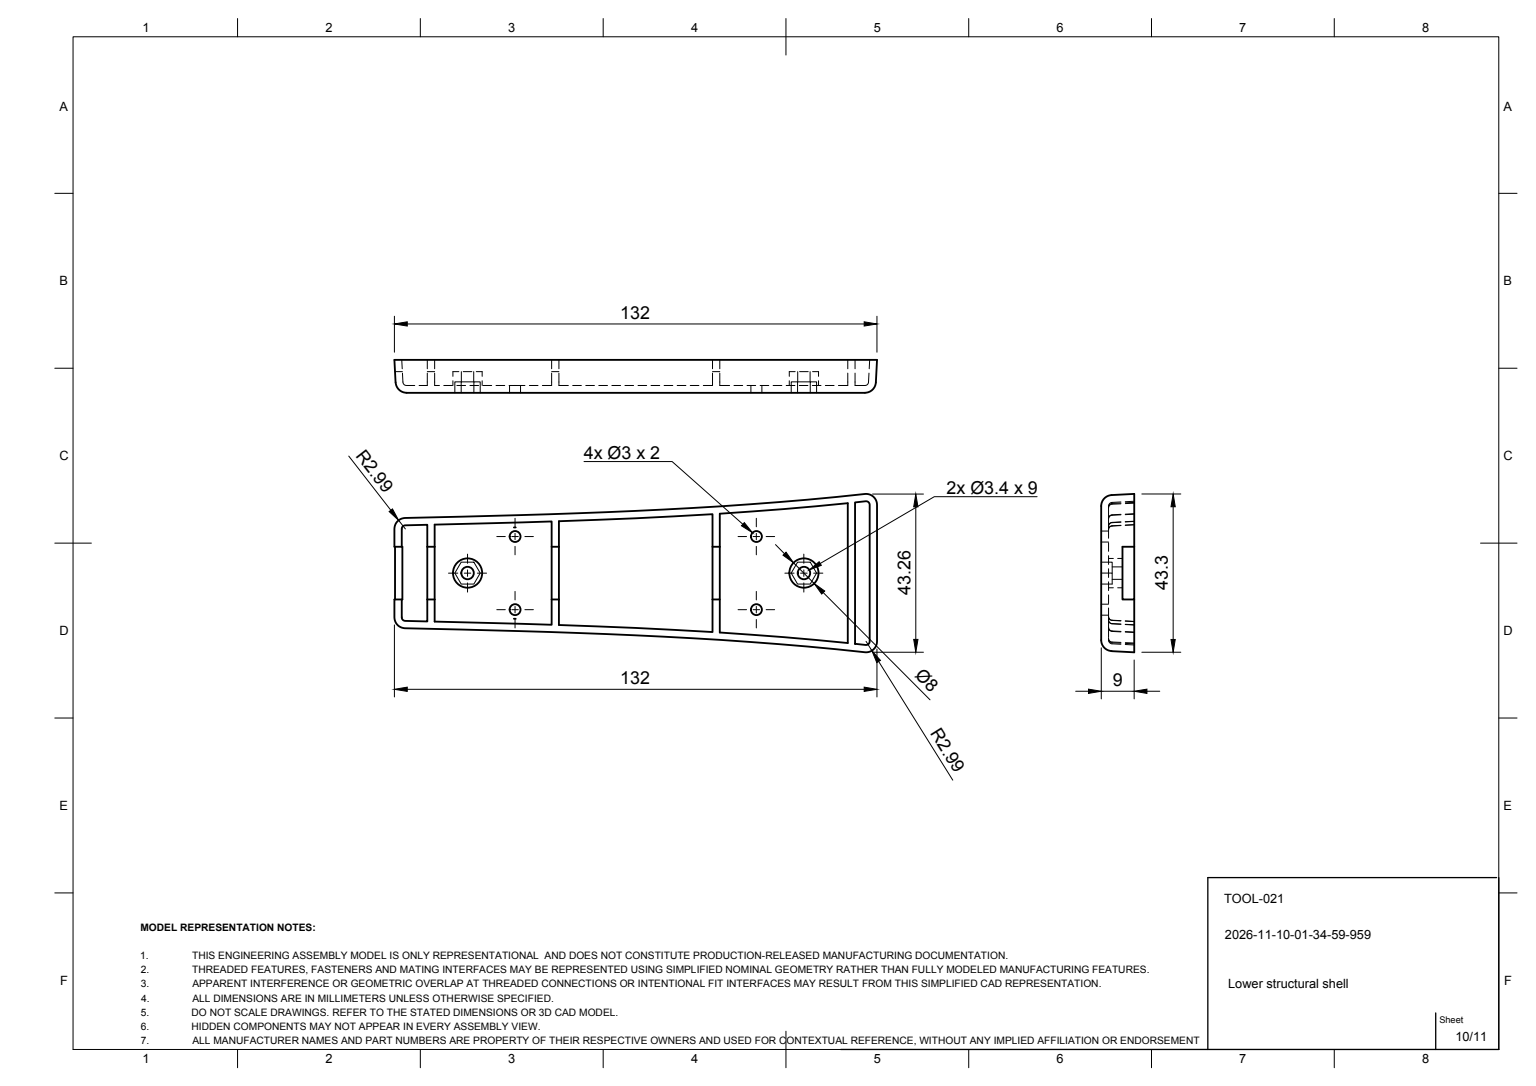
ISO-10303-21;
HEADER;
/* Generated by software containing ST-Developer
 * from STEP Tools, Inc. (www.steptools.com) 
 */

FILE_DESCRIPTION(
/* description */ (''),
/* implementation_level */ '2;1');

FILE_NAME(
/* name */ 'Lower structural shell.step',
/* time_stamp */ '2026-11-10T09:05:57-08:00',
/* author */ (''),
/* organization */ (''),
/* preprocessor_version */ 'ST-DEVELOPER v20.2',
/* originating_system */ 'Autodesk Translation Framework v15.17.0.0',
/* authorisation */ '');

FILE_SCHEMA (('AUTOMOTIVE_DESIGN { 1 0 10303 214 3 1 1 }'));
ENDSEC;

DATA;
#10=MECHANICAL_DESIGN_GEOMETRIC_PRESENTATION_REPRESENTATION('',(#570),#19618);
#83=SPHERICAL_SURFACE('',#7546,0.0999999999999999);
#84=SPHERICAL_SURFACE('',#7549,0.0999999999999997);
#85=SPHERICAL_SURFACE('',#7553,0.0999999999999998);
#86=SPHERICAL_SURFACE('',#7557,0.1);
#87=SPHERICAL_SURFACE('',#7562,0.3);
#88=SPHERICAL_SURFACE('',#7566,0.3);
#89=SPHERICAL_SURFACE('',#7570,0.3);
#90=SPHERICAL_SURFACE('',#7575,0.3);
#123=B_SPLINE_SURFACE_WITH_KNOTS('',3,3,((#12819,#12820,#12821,#12822),
(#12823,#12824,#12825,#12826),(#12827,#12828,#12829,#12830),(#12831,#12832,
#12833,#12834)),.UNSPECIFIED.,.F.,.F.,.F.,(4,4),(4,4),(0.0600191787356395,
0.326709122771036),(0.0105314009467253,0.683686938235975),.UNSPECIFIED.);
#124=B_SPLINE_SURFACE_WITH_KNOTS('',3,3,((#12839,#12840,#12841,#12842),
(#12843,#12844,#12845,#12846),(#12847,#12848,#12849,#12850),(#12851,#12852,
#12853,#12854)),.UNSPECIFIED.,.F.,.F.,.F.,(4,4),(4,4),(0.0251675824878611,
0.0470055662028096),(0.0103663370325175,0.682341693918943),
 .UNSPECIFIED.);
#125=B_SPLINE_SURFACE_WITH_KNOTS('',3,3,((#12864,#12865,#12866,#12867),
(#12868,#12869,#12870,#12871),(#12872,#12873,#12874,#12875),(#12876,#12877,
#12878,#12879),(#12880,#12881,#12882,#12883)),.UNSPECIFIED.,.F.,.F.,.F.,
(4,1,4),(4,4),(0.,0.571428571428571,1.),(0.796205213256333,4.31873271634551),
 .UNSPECIFIED.);
#126=B_SPLINE_SURFACE_WITH_KNOTS('',3,3,((#12888,#12889,#12890,#12891),
(#12892,#12893,#12894,#12895),(#12896,#12897,#12898,#12899),(#12900,#12901,
#12902,#12903),(#12904,#12905,#12906,#12907)),.UNSPECIFIED.,.F.,.F.,.F.,
(4,1,4),(4,4),(0.,0.571428571428571,1.),(0.335767855111383,0.605460332260614),
 .UNSPECIFIED.);
#127=B_SPLINE_SURFACE_WITH_KNOTS('',3,3,((#12926,#12927,#12928,#12929),
(#12930,#12931,#12932,#12933),(#12934,#12935,#12936,#12937),(#12938,#12939,
#12940,#12941),(#12942,#12943,#12944,#12945)),.UNSPECIFIED.,.F.,.F.,.F.,
(4,1,4),(4,4),(0.,0.571428571428571,1.),(8.8675541747208,12.3900816778099),
 .UNSPECIFIED.);
#128=B_SPLINE_SURFACE_WITH_KNOTS('',3,3,((#12950,#12951,#12952,#12953),
(#12954,#12955,#12956,#12957),(#12958,#12959,#12960,#12961),(#12962,#12963,
#12964,#12965)),.UNSPECIFIED.,.F.,.F.,.F.,(4,4),(4,4),(0.673290877228964,
0.939980821264432),(0.010531400969624,0.683686938235975),.UNSPECIFIED.);
#129=B_SPLINE_SURFACE_WITH_KNOTS('',3,3,((#12966,#12967,#12968,#12969),
(#12970,#12971,#12972,#12973),(#12974,#12975,#12976,#12977),(#12978,#12979,
#12980,#12981)),.UNSPECIFIED.,.F.,.F.,.F.,(4,4),(4,4),(0.952994433797115,
0.974832417512139),(0.0103663370325174,0.682341693895801),.UNSPECIFIED.);
#130=B_SPLINE_SURFACE_WITH_KNOTS('',3,3,((#13065,#13066,#13067,#13068),
(#13069,#13070,#13071,#13072),(#13073,#13074,#13075,#13076),(#13077,#13078,
#13079,#13080)),.UNSPECIFIED.,.F.,.F.,.F.,(4,4),(4,4),(0.341076481775573,
0.660379921919131),(0.0113804342297301,0.684288445414502),.UNSPECIFIED.);
#131=B_SPLINE_SURFACE_WITH_KNOTS('',3,3,((#13085,#13086,#13087,#13088),
(#13089,#13090,#13091,#13092),(#13093,#13094,#13095,#13096),(#13097,#13098,
#13099,#13100),(#13101,#13102,#13103,#13104)),.UNSPECIFIED.,.F.,.F.,.F.,
(4,1,4),(4,4),(0.,0.571428571428571,1.),(4.5128966022766,8.72381854299666),
 .UNSPECIFIED.);
#132=B_SPLINE_SURFACE_WITH_KNOTS('',3,3,((#13114,#13115,#13116,#13117),
(#13118,#13119,#13120,#13121),(#13122,#13123,#13124,#13125),(#13126,#13127,
#13128,#13129),(#13130,#13131,#13132,#13133)),.UNSPECIFIED.,.F.,.F.,.F.,
(4,1,4),(4,4),(0.,0.571428571428571,1.),(4.46246834806959,8.67339028878965),
 .UNSPECIFIED.);
#133=B_SPLINE_SURFACE_WITH_KNOTS('',3,3,((#13138,#13139,#13140,#13141),
(#13142,#13143,#13144,#13145),(#13146,#13147,#13148,#13149),(#13150,#13151,
#13152,#13153)),.UNSPECIFIED.,.F.,.F.,.F.,(4,4),(4,4),(0.33962007808087,
0.658923518224427),(0.0113804342297301,0.68428844541339),.UNSPECIFIED.);
#134=B_SPLINE_SURFACE_WITH_KNOTS('',3,3,((#13225,#13226,#13227,#13228),
(#13229,#13230,#13231,#13232),(#13233,#13234,#13235,#13236),(#13237,#13238,
#13239,#13240)),.UNSPECIFIED.,.F.,.F.,.F.,(4,4),(4,4),(0.67474627241906,
0.91907102854965),(0.0117551961069005,0.684448842095107),.UNSPECIFIED.);
#135=B_SPLINE_SURFACE_WITH_KNOTS('',3,3,((#13245,#13246,#13247,#13248),
(#13249,#13250,#13251,#13252),(#13253,#13254,#13255,#13256),(#13257,#13258,
#13259,#13260),(#13261,#13262,#13263,#13264)),.UNSPECIFIED.,.F.,.F.,.F.,
(4,1,4),(4,4),(0.,0.571428571428571,1.),(8.92068531110742,12.1251256661408),
 .UNSPECIFIED.);
#136=B_SPLINE_SURFACE_WITH_KNOTS('',3,3,((#13265,#13266,#13267,#13268),
(#13269,#13270,#13271,#13272),(#13273,#13274,#13275,#13276),(#13277,#13278,
#13279,#13280),(#13281,#13282,#13283,#13284)),.UNSPECIFIED.,.F.,.F.,.F.,
(4,1,4),(4,4),(0.,0.571428571428571,1.),(1.06116122492545,4.26560157995882),
 .UNSPECIFIED.);
#137=B_SPLINE_SURFACE_WITH_KNOTS('',3,3,((#13289,#13290,#13291,#13292),
(#13293,#13294,#13295,#13296),(#13297,#13298,#13299,#13300),(#13301,#13302,
#13303,#13304)),.UNSPECIFIED.,.F.,.F.,.F.,(4,4),(4,4),(0.0809289714503497,
0.325253727580939),(0.011755196108102,0.684448842095106),.UNSPECIFIED.);
#138=B_SPLINE_SURFACE_WITH_KNOTS('',3,3,((#13379,#13380,#13381,#13382),
(#13383,#13384,#13385,#13386),(#13387,#13388,#13389,#13390),(#13391,#13392,
#13393,#13394)),.UNSPECIFIED.,.F.,.F.,.F.,(4,4),(4,4),(0.932204931312898,
0.977820042778932),(0.0118590921259657,0.68448768567755),.UNSPECIFIED.);
#139=B_SPLINE_SURFACE_WITH_KNOTS('',3,3,((#13404,#13405,#13406,#13407),
(#13408,#13409,#13410,#13411),(#13412,#13413,#13414,#13415),(#13416,#13417,
#13418,#13419),(#13420,#13421,#13422,#13423)),.UNSPECIFIED.,.F.,.F.,.F.,
(4,1,4),(4,4),(0.,0.571428571428571,1.),(12.3228618033436,12.893479658151),
 .UNSPECIFIED.);
#140=B_SPLINE_SURFACE_WITH_KNOTS('',3,3,((#13437,#13438,#13439,#13440),
(#13441,#13442,#13443,#13444),(#13445,#13446,#13447,#13448),(#13449,#13450,
#13451,#13452)),.UNSPECIFIED.,.F.,.F.,.F.,(4,4),(4,4),(0.0221799572210682,
0.0677950686870383),(0.0118590921467069,0.68448768567755),.UNSPECIFIED.);
#141=B_SPLINE_SURFACE_WITH_KNOTS('',3,3,((#13462,#13463,#13464,#13465),
(#13466,#13467,#13468,#13469),(#13470,#13471,#13472,#13473),(#13474,#13475,
#13476,#13477),(#13478,#13479,#13480,#13481)),.UNSPECIFIED.,.F.,.F.,.F.,
(4,1,4),(4,4),(0.,0.571428571428571,1.),(0.29280723291527,0.863425087722636),
 .UNSPECIFIED.);
#142=B_SPLINE_SURFACE_WITH_KNOTS('',3,3,((#13495,#13496,#13497,#13498),
(#13499,#13500,#13501,#13502),(#13503,#13504,#13505,#13506),(#13507,#13508,
#13509,#13510),(#13511,#13512,#13513,#13514)),.UNSPECIFIED.,.F.,.F.,.F.,
(4,1,4),(4,4),(0.,0.571428571428571,1.),(0.00866835330220971,0.617725317592517),
 .UNSPECIFIED.);
#143=B_SPLINE_SURFACE_WITH_KNOTS('',3,3,((#13521,#13522,#13523,#13524),
(#13525,#13526,#13527,#13528),(#13529,#13530,#13531,#13532),(#13533,#13534,
#13535,#13536),(#13537,#13538,#13539,#13540),(#13541,#13542,#13543,#13544)),
 .UNSPECIFIED.,.F.,.F.,.F.,(4,1,1,4),(4,4),(0.,0.285714285714286,0.571428571428571,
1.),(0.00654045782928703,0.615688454110788),.UNSPECIFIED.);
#144=B_SPLINE_SURFACE_WITH_KNOTS('',3,3,((#13549,#13550,#13551,#13552),
(#13553,#13554,#13555,#13556),(#13557,#13558,#13559,#13560),(#13561,#13562,
#13563,#13564),(#13565,#13566,#13567,#13568),(#13569,#13570,#13571,#13572)),
 .UNSPECIFIED.,.F.,.F.,.F.,(4,1,1,4),(4,4),(0.,0.285714285714286,0.571428571428571,
1.),(0.00659363931523289,0.615688454110787),.UNSPECIFIED.);
#145=B_SPLINE_SURFACE_WITH_KNOTS('',3,3,((#13577,#13578,#13579,#13580),
(#13581,#13582,#13583,#13584),(#13585,#13586,#13587,#13588),(#13589,#13590,
#13591,#13592),(#13593,#13594,#13595,#13596)),.UNSPECIFIED.,.F.,.F.,.F.,
(4,1,4),(4,4),(0.,0.571428571428571,1.),(12.5808265588057,12.8505190359549),
 .UNSPECIFIED.);
#146=B_SPLINE_SURFACE_WITH_KNOTS('',3,3,((#13597,#13598,#13599,#13600),
(#13601,#13602,#13603,#13604),(#13605,#13606,#13607,#13608),(#13609,#13610,
#13611,#13612),(#13613,#13614,#13615,#13616)),.UNSPECIFIED.,.F.,.F.,.F.,
(4,1,4),(4,4),(0.,0.571428571428571,1.),(0.00865878607617127,0.617725317592517),
 .UNSPECIFIED.);
#147=B_SPLINE_SURFACE_WITH_KNOTS('',3,3,((#13642,#13643,#13644,#13645),
(#13646,#13647,#13648,#13649),(#13650,#13651,#13652,#13653),(#13654,#13655,
#13656,#13657),(#13658,#13659,#13660,#13661)),.UNSPECIFIED.,.F.,.F.,.F.,
(4,1,4),(4,4),(0.,0.571428571428571,1.),(-0.00615755989250974,0.617725317592517),
 .UNSPECIFIED.);
#148=B_SPLINE_SURFACE_WITH_KNOTS('',3,3,((#13680,#13681,#13682,#13683,#13684),
(#13685,#13686,#13687,#13688,#13689),(#13690,#13691,#13692,#13693,#13694),
(#13695,#13696,#13697,#13698,#13699),(#13700,#13701,#13702,#13703,#13704)),
 .UNSPECIFIED.,.F.,.F.,.F.,(4,1,4),(4,1,4),(0.,0.571428571428571,1.),(0.335767855111383,
5.71764434212835,12.893479658151),.UNSPECIFIED.);
#149=B_SPLINE_SURFACE_WITH_KNOTS('',3,3,((#13715,#13716,#13717,#13718),
(#13719,#13720,#13721,#13722),(#13723,#13724,#13725,#13726),(#13727,#13728,
#13729,#13730),(#13731,#13732,#13733,#13734),(#13735,#13736,#13737,#13738)),
 .UNSPECIFIED.,.F.,.F.,.F.,(4,1,1,4),(4,4),(0.,0.285714285714286,0.571428571428571,
1.),(-0.00844595120920508,0.615688454110788),.UNSPECIFIED.);
#150=B_SPLINE_SURFACE_WITH_KNOTS('',3,3,((#13747,#13748,#13749,#13750),
(#13751,#13752,#13753,#13754),(#13755,#13756,#13757,#13758),(#13759,#13760,
#13761,#13762),(#13763,#13764,#13765,#13766),(#13767,#13768,#13769,#13770)),
 .UNSPECIFIED.,.F.,.F.,.F.,(4,1,1,4),(4,4),(0.,0.285714285714286,0.571428571428571,
1.),(-0.00828643285111643,0.615688454110787),.UNSPECIFIED.);
#151=B_SPLINE_SURFACE_WITH_KNOTS('',3,3,((#13779,#13780,#13781,#13782,#13783),
(#13784,#13785,#13786,#13787,#13788),(#13789,#13790,#13791,#13792,#13793),
(#13794,#13795,#13796,#13797,#13798),(#13799,#13800,#13801,#13802,#13803)),
 .UNSPECIFIED.,.F.,.F.,.F.,(4,1,4),(4,1,4),(0.,0.571428571428571,1.),(0.29280723291527,
7.4686425489379,12.8505190359549),.UNSPECIFIED.);
#152=B_SPLINE_SURFACE_WITH_KNOTS('',3,3,((#13814,#13815,#13816,#13817),
(#13818,#13819,#13820,#13821),(#13822,#13823,#13824,#13825),(#13826,#13827,
#13828,#13829),(#13830,#13831,#13832,#13833)),.UNSPECIFIED.,.F.,.F.,.F.,
(4,1,4),(4,4),(0.,0.571428571428571,1.),(-0.0061862132014275,0.617725317592517),
 .UNSPECIFIED.);
#153=B_SPLINE_SURFACE_WITH_KNOTS('',3,3,((#13842,#13843,#13844,#13845),
(#13846,#13847,#13848,#13849),(#13850,#13851,#13852,#13853),(#13854,#13855,
#13856,#13857)),.UNSPECIFIED.,.F.,.F.,.F.,(4,4),(4,4),(0.025165545222094,
0.977821881680028),(0.,0.68448768567755),.UNSPECIFIED.);
#154=B_SPLINE_SURFACE_WITH_KNOTS('',3,3,((#13860,#13861,#13862,#13863),
(#13864,#13865,#13866,#13867),(#13868,#13869,#13870,#13871),(#13872,#13873,
#13874,#13875)),.UNSPECIFIED.,.F.,.F.,.F.,(4,4),(4,4),(0.0221781183199723,
0.974834454777906),(0.,0.68448768567755),.UNSPECIFIED.);
#267=B_SPLINE_CURVE_WITH_KNOTS('',3,(#11773,#11774,#11775,#11776),
 .UNSPECIFIED.,.F.,.F.,(4,4),(3.28016616408593,4.26236080300681),
 .UNSPECIFIED.);
#268=B_SPLINE_CURVE_WITH_KNOTS('',3,(#11780,#11781,#11782,#11783),
 .UNSPECIFIED.,.F.,.F.,(4,4),(8.92392608805945,9.90612072688831),
 .UNSPECIFIED.);
#269=B_SPLINE_CURVE_WITH_KNOTS('',3,(#11785,#11786,#11787,#11788,#11789,
#11790,#11791,#11792,#11793,#11794,#11795,#11796,#11797,#11798,#11799,#11800,
#11801,#11802,#11803),.UNSPECIFIED.,.F.,.F.,(4,3,3,3,3,3,4),(-0.050768112872884,
-0.0388528786649772,-0.0311058171716578,-0.0259830388669653,-0.0210744122964195,
-0.0143837148934404,0.),.UNSPECIFIED.);
#270=B_SPLINE_CURVE_WITH_KNOTS('',3,(#11805,#11806,#11807,#11808),
 .UNSPECIFIED.,.F.,.F.,(4,4),(9.9568018127159,12.1251256661408),
 .UNSPECIFIED.);
#271=B_SPLINE_CURVE_WITH_KNOTS('',3,(#11812,#11813,#11814,#11815),
 .UNSPECIFIED.,.F.,.F.,(4,4),(1.06116122492545,3.22948508825557),
 .UNSPECIFIED.);
#272=B_SPLINE_CURVE_WITH_KNOTS('',3,(#11816,#11817,#11818,#11819,#11820,
#11821,#11822,#11823,#11824,#11825,#11826,#11827,#11828,#11829,#11830,#11831,
#11832,#11833,#11834),.UNSPECIFIED.,.F.,.F.,(4,3,3,3,3,3,4),(-0.0507681129736439,
-0.0388528772897764,-0.0311058147321604,-0.0259830361493327,-0.0210744097201194,
-0.0143837130754026,-9.90506278315E-9),.UNSPECIFIED.);
#273=B_SPLINE_CURVE_WITH_KNOTS('',3,(#12042,#12043,#12044,#12045,#12046,
#12047),.UNSPECIFIED.,.F.,.F.,(4,2,4),(-0.605566356596631,-0.303329629920269,
-0.000148729590407126),.UNSPECIFIED.);
#274=B_SPLINE_CURVE_WITH_KNOTS('',3,(#12049,#12050,#12051,#12052,#12053,
#12054,#12055,#12056,#12057,#12058,#12059,#12060,#12061,#12062,#12063,#12064,
#12065,#12066,#12067,#12068,#12069,#12070,#12071,#12072,#12073,#12074,#12075,
#12076),.UNSPECIFIED.,.F.,.F.,(4,3,3,3,3,3,3,3,3,4),(-0.153210533292091,
-0.129383071834804,-0.117098895005168,-0.0931297672424715,-0.0778761857300216,
-0.065564095006876,-0.0417435583396367,-0.038874550231651,-0.0150983388519663,
0.),.UNSPECIFIED.);
#275=B_SPLINE_CURVE_WITH_KNOTS('',3,(#12080,#12081,#12082,#12083,#12084,
#12085,#12086,#12087,#12088,#12089,#12090,#12091,#12092,#12093,#12094,#12095,
#12096,#12097,#12098,#12099,#12100,#12101,#12102,#12103,#12104,#12105,#12106,
#12107),.UNSPECIFIED.,.F.,.F.,(4,3,3,3,3,3,3,3,3,4),(-0.153244081227051,
-0.129493605146206,-0.117970006482883,-0.0941492904140308,-0.0876825809854227,
-0.078828741443105,-0.0548877675055393,-0.0394694906046094,-0.0155984926894347,
0.),.UNSPECIFIED.);
#276=B_SPLINE_CURVE_WITH_KNOTS('',3,(#12108,#12109,#12110,#12111,#12112,
#12113),.UNSPECIFIED.,.F.,.F.,(4,2,4),(-0.606539490527658,-0.303329031627741,
-0.00112184825655631),.UNSPECIFIED.);
#277=B_SPLINE_CURVE_WITH_KNOTS('',3,(#12118,#12119,#12120,#12121,#12122,
#12123),.UNSPECIFIED.,.F.,.F.,(4,2,4),(-0.606785247764818,-0.303663188081886,
-0.00088649083675002),.UNSPECIFIED.);
#278=B_SPLINE_CURVE_WITH_KNOTS('',3,(#12125,#12126,#12127,#12128,#12129,
#12130,#12131,#12132,#12133,#12134,#12135,#12136,#12137,#12138,#12139,#12140,
#12141,#12142,#12143,#12144,#12145,#12146,#12147,#12148,#12149,#12150,#12151,
#12152),.UNSPECIFIED.,.F.,.F.,(4,3,3,3,3,3,3,3,3,4),(-0.15258577077829,
-0.128839317352572,-0.117158786685373,-0.0932148261566644,-0.0780319390000633,
-0.0653676349965338,-0.0415665498371782,-0.0389909618069961,-0.0152059030050533,
0.),.UNSPECIFIED.);
#279=B_SPLINE_CURVE_WITH_KNOTS('',3,(#12156,#12157,#12158,#12159,#12160,
#12161,#12162,#12163,#12164,#12165,#12166,#12167,#12168,#12169,#12170,#12171,
#12172,#12173,#12174,#12175,#12176,#12177,#12178,#12179,#12180,#12181,#12182,
#12183),.UNSPECIFIED.,.F.,.F.,(4,3,3,3,3,3,3,3,3,4),(-0.152596853546747,
-0.128825864440686,-0.115507515430042,-0.0917263797372463,-0.0872428123353572,
-0.0783995504057471,-0.0544835945915644,-0.0392209901554083,-0.0154275313391792,
0.),.UNSPECIFIED.);
#280=B_SPLINE_CURVE_WITH_KNOTS('',3,(#12185,#12186,#12187,#12188,#12189,
#12190),.UNSPECIFIED.,.F.,.F.,(4,2,4),(-0.606440835737524,-0.303663090452391,
-0.000542069086802599),.UNSPECIFIED.);
#281=B_SPLINE_CURVE_WITH_KNOTS('',3,(#12196,#12197,#12198,#12199,#12200,
#12201),.UNSPECIFIED.,.F.,.F.,(4,2,4),(-0.607379220946441,-0.303761646676304,
-0.00124422999587004),.UNSPECIFIED.);
#282=B_SPLINE_CURVE_WITH_KNOTS('',3,(#12203,#12204,#12205,#12206,#12207,
#12208,#12209,#12210,#12211,#12212,#12213,#12214,#12215,#12216,#12217,#12218,
#12219,#12220,#12221,#12222,#12223,#12224,#12225,#12226,#12227,#12228,#12229,
#12230),.UNSPECIFIED.,.F.,.F.,(4,3,3,3,3,3,3,3,3,4),(-0.152287640102895,
-0.128554450486317,-0.115193035178751,-0.0912770810520543,-0.0781028969167454,
-0.0652733399726575,-0.0414820896655672,-0.0390446621366508,-0.0152552334863041,
0.),.UNSPECIFIED.);
#283=B_SPLINE_CURVE_WITH_KNOTS('',3,(#12234,#12235,#12236,#12237,#12238,
#12239,#12240,#12241,#12242,#12243,#12244,#12245,#12246,#12247,#12248,#12249,
#12250,#12251,#12252,#12253,#12254,#12255,#12256,#12257,#12258,#12259,#12260,
#12261),.UNSPECIFIED.,.F.,.F.,(4,3,3,3,3,3,3,3,3,4),(-0.152291020205185,
-0.128517753946702,-0.115248901231919,-0.0914807886786037,-0.0870359119466785,
-0.0782017654295232,-0.054298407767766,-0.03910658747416,-0.0153486482327859,
0.),.UNSPECIFIED.);
#284=B_SPLINE_CURVE_WITH_KNOTS('',3,(#12263,#12264,#12265,#12266,#12267,
#12268),.UNSPECIFIED.,.F.,.F.,(4,2,4),(-0.606279550122448,-0.303761677523001,
-0.000144559171857295),.UNSPECIFIED.);
#285=B_SPLINE_CURVE_WITH_KNOTS('',3,(#12274,#12275,#12276,#12277,#12278,
#12279),.UNSPECIFIED.,.F.,.F.,(4,2,4),(-0.607536685592867,-0.303784463250135,
-0.00133982193348342),.UNSPECIFIED.);
#286=B_SPLINE_CURVE_WITH_KNOTS('',3,(#12280,#12281,#12282,#12283,#12284,
#12285,#12286,#12287,#12288,#12289,#12290,#12291,#12292,#12293,#12294,#12295,
#12296,#12297,#12298,#12299,#12300,#12301,#12302,#12303,#12304,#12305,#12306,
#12307),.UNSPECIFIED.,.F.,.F.,(4,3,3,3,3,3,3,3,3,4),(-0.152217684890348,
-0.128490376540845,-0.11516578527262,-0.091253137134092,-0.0781160865160423,
-0.0652495101170982,-0.0414606291875136,-0.0390546905501479,-0.015263466236765,
0.),.UNSPECIFIED.);
#287=B_SPLINE_CURVE_WITH_KNOTS('',3,(#12309,#12310,#12311,#12312,#12313,
#12314,#12315,#12316,#12317,#12318,#12319,#12320,#12321,#12322,#12323,#12324,
#12325,#12326,#12327,#12328,#12329,#12330,#12331,#12332,#12333,#12334,#12335,
#12336),.UNSPECIFIED.,.F.,.F.,(4,3,3,3,3,3,3,3,3,4),(-0.152219351639196,
-0.128444680332832,-0.115193337419806,-0.0914284185691762,-0.0869890032859244,
-0.0781648487722283,-0.0542647883944502,-0.0390852411900305,-0.0153331469286526,
0.),.UNSPECIFIED.);
#288=B_SPLINE_CURVE_WITH_KNOTS('',3,(#12338,#12339,#12340,#12341,#12342,
#12343),.UNSPECIFIED.,.F.,.F.,(4,2,4),(-0.606231877025315,-0.303784501204342,
-3.50089943914611E-5),.UNSPECIFIED.);
#289=B_SPLINE_CURVE_WITH_KNOTS('',3,(#12349,#12350,#12351,#12352),
 .UNSPECIFIED.,.F.,.F.,(4,4),(0.0108333608245492,0.617725317592517),
 .UNSPECIFIED.);
#290=B_SPLINE_CURVE_WITH_KNOTS('',3,(#12356,#12357,#12358,#12359),
 .UNSPECIFIED.,.F.,.F.,(4,4),(-0.617725317592517,-0.0108333608245492),
 .UNSPECIFIED.);
#291=B_SPLINE_CURVE_WITH_KNOTS('',3,(#12362,#12363,#12364,#12365),
 .UNSPECIFIED.,.F.,.F.,(4,4),(8.65483889175297,12.1899094612697),
 .UNSPECIFIED.);
#292=B_SPLINE_CURVE_WITH_KNOTS('',3,(#12366,#12367,#12368,#12369),
 .UNSPECIFIED.,.F.,.F.,(4,4),(0.491886782059505,4.00844302274363),
 .UNSPECIFIED.);
#293=B_SPLINE_CURVE_WITH_KNOTS('',3,(#12372,#12373,#12374,#12375,#12376,
#12377,#12378,#12379,#12380,#12381),.UNSPECIFIED.,.F.,.F.,(4,3,3,4),(4.20909064274042,
6.3236533433415,8.26419514194387,8.41669725637478),.UNSPECIFIED.);
#294=B_SPLINE_CURVE_WITH_KNOTS('',3,(#12384,#12385,#12386,#12387),
 .UNSPECIFIED.,.F.,.F.,(4,4),(8.61714174069208,11.8187712274298),
 .UNSPECIFIED.);
#295=B_SPLINE_CURVE_WITH_KNOTS('',3,(#12391,#12392,#12393,#12394),
 .UNSPECIFIED.,.F.,.F.,(4,4),(12.0182076143484,12.6179302061492),
 .UNSPECIFIED.);
#296=B_SPLINE_CURVE_WITH_KNOTS('',3,(#12395,#12396,#12397,#12398,#12399,
#12400,#12401,#12402,#12403,#12404,#12405,#12406,#12407,#12408,#12409,#12410,
#12411,#12412,#12413,#12414,#12415,#12416,#12417,#12418,#12419,#12420,#12421,
#12422),.UNSPECIFIED.,.F.,.F.,(4,3,3,3,3,3,3,3,3,4),(0.,0.023812730958415,
0.0390943730497349,0.0628727645281949,0.0664866407211859,0.0780895647789142,
0.102003044086093,0.117056568347941,0.14081843048439,0.155095961761698),
 .UNSPECIFIED.);
#297=B_SPLINE_CURVE_WITH_KNOTS('',3,(#12426,#12427,#12428,#12429,#12430,
#12431,#12432,#12433,#12434,#12435,#12436,#12437,#12438,#12439,#12440,#12441,
#12442,#12443,#12444,#12445,#12446,#12447,#12448,#12449,#12450,#12451,#12452,
#12453,#12454,#12455,#12456,#12457,#12458,#12459,#12460,#12461,#12462),
 .UNSPECIFIED.,.F.,.F.,(4,3,3,3,3,3,3,3,3,3,3,3,4),(0.,0.0535193130531386,
0.107740084455895,0.117281563739951,0.171478196787188,0.199460035548543,
0.234266327019636,0.287962832542679,0.34249270416273,0.351167719367162,
0.408228095477446,0.46132246935065,0.46528847158773),.UNSPECIFIED.);
#298=B_SPLINE_CURVE_WITH_KNOTS('',3,(#12464,#12465,#12466,#12467),
 .UNSPECIFIED.,.F.,.F.,(4,4),(0.0221781183199723,0.974834454777906),
 .UNSPECIFIED.);
#299=B_SPLINE_CURVE_WITH_KNOTS('',3,(#12469,#12470,#12471,#12472,#12473,
#12474,#12475,#12476,#12477,#12478,#12479,#12480,#12481,#12482,#12483,#12484,
#12485,#12486,#12487,#12488,#12489,#12490,#12491,#12492,#12493,#12494,#12495,
#12496,#12497,#12498,#12499,#12500,#12501,#12502,#12503,#12504,#12505,#12506,
#12507,#12508,#12509,#12510,#12511),.UNSPECIFIED.,.F.,.F.,(4,3,3,3,3,3,
3,3,3,3,3,3,3,3,4),(0.,0.0533317239385299,0.107762434368039,0.117305236535198,
0.171635266834242,0.216430402805854,0.234303130921432,0.288010415584935,
0.341932185058889,0.351200358601802,0.360578786332496,0.414653942238971,
0.427906071157934,0.482008506259547,0.504658879840573),.UNSPECIFIED.);
#300=B_SPLINE_CURVE_WITH_KNOTS('',3,(#12515,#12516,#12517,#12518,#12519,
#12520,#12521,#12522,#12523,#12524,#12525,#12526,#12527,#12528,#12529,#12530,
#12531,#12532,#12533,#12534,#12535,#12536,#12537,#12538,#12539,#12540,#12541,
#12542,#12543,#12544,#12545,#12546,#12547,#12548,#12549,#12550,#12551,#12552,
#12553,#12554,#12555,#12556,#12557),.UNSPECIFIED.,.F.,.F.,(4,3,3,3,3,3,
3,3,3,3,3,3,3,3,4),(0.,0.0533492049661439,0.107791770949794,0.117401360885473,
0.171729175646356,0.216477851539682,0.234467324023732,0.288191829779795,
0.342104640447882,0.351366010290958,0.360619117109406,0.414688080797906,
0.427993719046535,0.482081475021072,0.504664253934307),.UNSPECIFIED.);
#301=B_SPLINE_CURVE_WITH_KNOTS('',3,(#12559,#12560,#12561,#12562),
 .UNSPECIFIED.,.F.,.F.,(4,4),(0.0251655452220943,0.977821881680028),
 .UNSPECIFIED.);
#302=B_SPLINE_CURVE_WITH_KNOTS('',3,(#12564,#12565,#12566,#12567,#12568,
#12569,#12570,#12571,#12572,#12573,#12574,#12575,#12576,#12577,#12578,#12579,
#12580,#12581,#12582,#12583,#12584,#12585,#12586,#12587,#12588,#12589,#12590,
#12591,#12592,#12593,#12594,#12595,#12596,#12597,#12598,#12599,#12600),
 .UNSPECIFIED.,.F.,.F.,(4,3,3,3,3,3,3,3,3,3,3,3,4),(0.,0.053523079491772,
0.107745541051727,0.117301531762597,0.171497090450284,0.19946878868074,
0.234298606923062,0.287998861062908,0.34252758042597,0.351197710209308,
0.408243668718811,0.4613343165756,0.465289627228313),.UNSPECIFIED.);
#303=B_SPLINE_CURVE_WITH_KNOTS('',3,(#12603,#12604,#12605,#12606,#12607,
#12608,#12609,#12610,#12611,#12612,#12613,#12614,#12615,#12616,#12617,#12618,
#12619,#12620,#12621,#12622,#12623,#12624,#12625,#12626,#12627,#12628,#12629,
#12630),.UNSPECIFIED.,.F.,.F.,(4,3,3,3,3,3,3,3,3,4),(0.,0.0238139464176845,
0.039101051769884,0.0628789982206146,0.0664894862143964,0.0781003874493316,
0.102014483019035,0.11706667068295,0.140827139970411,0.155096347075245),
 .UNSPECIFIED.);
#304=B_SPLINE_CURVE_WITH_KNOTS('',3,(#12632,#12633,#12634,#12635),
 .UNSPECIFIED.,.F.,.F.,(4,4),(2.42791692093292E-5,0.602904494019558),
 .UNSPECIFIED.);
#305=B_SPLINE_CURVE_WITH_KNOTS('',3,(#12638,#12639,#12640,#12641),
 .UNSPECIFIED.,.F.,.F.,(4,4),(0.8033909285608,4.02187648095927),
 .UNSPECIFIED.);
#306=B_SPLINE_CURVE_WITH_KNOTS('',3,(#12644,#12645,#12646,#12647,#12648,
#12649,#12650,#12651,#12652,#12653),.UNSPECIFIED.,.F.,.F.,(4,3,3,4),(4.22337623295021,
6.17414866693447,6.32726315261627,8.45313487255185),.UNSPECIFIED.);
#307=B_SPLINE_CURVE_WITH_KNOTS('',3,(#12657,#12658,#12659,#12660),
 .UNSPECIFIED.,.F.,.F.,(4,4),(12.3921295467468,12.6843586902602),
 .UNSPECIFIED.);
#308=B_SPLINE_CURVE_WITH_KNOTS('',3,(#12662,#12663,#12664,#12665,#12666,
#12667,#12668,#12669,#12670,#12671,#12672,#12673,#12674,#12675,#12676,#12677,
#12678,#12679,#12680,#12681,#12682,#12683,#12684,#12685,#12686,#12687,#12688,
#12689,#12690,#12691,#12692,#12693,#12694,#12695),.UNSPECIFIED.,.F.,.F.,
(4,3,3,3,3,3,3,3,3,3,3,4),(0.,0.0238043957114055,0.0391346151758438,0.0629652053320384,
0.0721593756253901,0.0781571886687045,0.101948185591131,0.117123476992186,
0.12020682003633,0.142665945482357,0.166389927689249,0.168222194312373),
 .UNSPECIFIED.);
#309=B_SPLINE_CURVE_WITH_KNOTS('',3,(#12699,#12700,#12701,#12702,#12703,
#12704,#12705,#12706,#12707,#12708,#12709,#12710,#12711,#12712,#12713,#12714,
#12715,#12716,#12717,#12718,#12719,#12720,#12721,#12722,#12723,#12724,#12725,
#12726,#12727,#12728,#12729,#12730,#12731,#12732),.UNSPECIFIED.,.F.,.F.,
(4,3,3,3,3,3,3,3,3,3,3,4),(0.,0.023797882907907,0.039102479174454,0.0629340675289177,
0.0721439954475325,0.0781021576199648,0.101891255326939,0.117067721419617,
0.120193732390416,0.142636523050355,0.16636673084783,0.168220399847748),
 .UNSPECIFIED.);
#310=B_SPLINE_CURVE_WITH_KNOTS('',3,(#12734,#12735,#12736,#12737),
 .UNSPECIFIED.,.F.,.F.,(4,4),(2.71213177756024E-5,0.290725780256064),
 .UNSPECIFIED.);
#311=B_SPLINE_CURVE_WITH_KNOTS('',3,(#12747,#12748,#12749,#12750,#12751,
#12752),.UNSPECIFIED.,.F.,.F.,(4,2,4),(-0.6065913737563,-0.303324265158378,
-0.00121210420063977),.UNSPECIFIED.);
#312=B_SPLINE_CURVE_WITH_KNOTS('',3,(#12754,#12755,#12756,#12757,#12758,
#12759),.UNSPECIFIED.,.F.,.F.,(4,2,4),(-0.605468679705391,-0.303324901248498,
-8.9425867424664E-5),.UNSPECIFIED.);
#313=B_SPLINE_CURVE_WITH_KNOTS('',3,(#12761,#12762,#12763,#12764,#12765,
#12766,#12767,#12768,#12769,#12770,#12771,#12772,#12773,#12774,#12775,#12776,
#12777,#12778,#12779,#12780,#12781,#12782,#12783,#12784,#12785,#12786,#12787,
#12788),.UNSPECIFIED.,.F.,.F.,(4,3,3,3,3,3,3,3,3,4),(-0.153261590805415,
-0.129427422483982,-0.117093626371441,-0.093122524304512,-0.077863059046492,
-0.0655799937729104,-0.0417579003169496,-0.0388648221790391,-0.0150894148558222,
0.),.UNSPECIFIED.);
#314=B_SPLINE_CURVE_WITH_KNOTS('',3,(#12791,#12792,#12793,#12794,#12795,
#12796,#12797,#12798,#12799,#12800,#12801,#12802,#12803,#12804,#12805,#12806,
#12807,#12808,#12809,#12810,#12811,#12812,#12813,#12814,#12815,#12816,#12817,
#12818),.UNSPECIFIED.,.F.,.F.,(4,3,3,3,3,3,3,3,3,4),(-0.153296867786173,
-0.129546774976449,-0.118009772088948,-0.0941871764575653,-0.08771862273971,
-0.0788646444725944,-0.0549216410880561,-0.0394902966566095,-0.0156128557692252,
0.),.UNSPECIFIED.);
#315=B_SPLINE_CURVE_WITH_KNOTS('',3,(#12835,#12836,#12837,#12838),
 .UNSPECIFIED.,.F.,.F.,(4,4),(-4.3123055228435,-0.796205213256333),
 .UNSPECIFIED.);
#316=B_SPLINE_CURVE_WITH_KNOTS('',3,(#12856,#12857,#12858,#12859),
 .UNSPECIFIED.,.F.,.F.,(4,4),(-0.594853877716395,-0.335767855111383),
 .UNSPECIFIED.);
#317=B_SPLINE_CURVE_WITH_KNOTS('',3,(#12860,#12861,#12862,#12863),
 .UNSPECIFIED.,.F.,.F.,(4,4),(-0.615688454110788,-0.00935595183171186),
 .UNSPECIFIED.);
#318=B_SPLINE_CURVE_WITH_KNOTS('',3,(#12884,#12885,#12886,#12887),
 .UNSPECIFIED.,.F.,.F.,(4,4),(0.806548880270408,4.31873271634551),
 .UNSPECIFIED.);
#319=B_SPLINE_CURVE_WITH_KNOTS('',3,(#12909,#12910,#12911,#12912),
 .UNSPECIFIED.,.F.,.F.,(4,4),(0.335767855111383,0.605460332260614),
 .UNSPECIFIED.);
#320=B_SPLINE_CURVE_WITH_KNOTS('',3,(#12915,#12916,#12917,#12918),
 .UNSPECIFIED.,.F.,.F.,(4,4),(8.8675541747208,12.379738010796),
 .UNSPECIFIED.);
#321=B_SPLINE_CURVE_WITH_KNOTS('',3,(#12921,#12922,#12923,#12924),
 .UNSPECIFIED.,.F.,.F.,(4,4),(12.5808265588057,12.8505190359549),
 .UNSPECIFIED.);
#322=B_SPLINE_CURVE_WITH_KNOTS('',3,(#12946,#12947,#12948,#12949),
 .UNSPECIFIED.,.F.,.F.,(4,4),(-12.3900816778099,-8.87398136822274),
 .UNSPECIFIED.);
#323=B_SPLINE_CURVE_WITH_KNOTS('',3,(#12983,#12984,#12985,#12986),
 .UNSPECIFIED.,.F.,.F.,(4,4),(0.00935595183171174,0.615688454110787),
 .UNSPECIFIED.);
#324=B_SPLINE_CURVE_WITH_KNOTS('',3,(#12987,#12988,#12989,#12990),
 .UNSPECIFIED.,.F.,.F.,(4,4),(-12.8505190359549,-12.5914330133498),
 .UNSPECIFIED.);
#325=B_SPLINE_CURVE_WITH_KNOTS('',3,(#12993,#12994,#12995,#12996,#12997,
#12998),.UNSPECIFIED.,.F.,.F.,(4,2,4),(-0.606830654194234,-0.303665168982051,
-0.00091389508118378),.UNSPECIFIED.);
#326=B_SPLINE_CURVE_WITH_KNOTS('',3,(#13000,#13001,#13002,#13003,#13004,
#13005,#13006,#13007,#13008,#13009,#13010,#13011,#13012,#13013,#13014,#13015,
#13016,#13017,#13018,#13019,#13020,#13021,#13022,#13023,#13024,#13025,#13026,
#13027),.UNSPECIFIED.,.F.,.F.,(4,3,3,3,3,3,3,3,3,4),(-0.152562937837783,
-0.12881903955137,-0.117160811640917,-0.0932181166800446,-0.0780374575565173,
-0.0653603882662585,-0.0415602279441365,-0.0389951227734853,-0.0152093108541457,
0.),.UNSPECIFIED.);
#327=B_SPLINE_CURVE_WITH_KNOTS('',3,(#13031,#13032,#13033,#13034,#13035,
#13036,#13037,#13038,#13039,#13040,#13041,#13042,#13043,#13044,#13045,#13046,
#13047,#13048,#13049,#13050,#13051,#13052,#13053,#13054,#13055,#13056,#13057,
#13058),.UNSPECIFIED.,.F.,.F.,(4,3,3,3,3,3,3,3,3,4),(-0.152573286042523,
-0.128801685906155,-0.115487540236632,-0.091707628219999,-0.0872268515824704,
-0.07838422198738,-0.0544695788315335,-0.0392121213631617,-0.0154211067806385,
0.),.UNSPECIFIED.);
#328=B_SPLINE_CURVE_WITH_KNOTS('',3,(#13059,#13060,#13061,#13062,#13063,
#13064),.UNSPECIFIED.,.F.,.F.,(4,2,4),(-0.606417229744719,-0.30366508312326,
-0.000500462001714608),.UNSPECIFIED.);
#329=B_SPLINE_CURVE_WITH_KNOTS('',3,(#13081,#13082,#13083,#13084),
 .UNSPECIFIED.,.F.,.F.,(4,4),(-8.7204856127415,-4.5128966022766),
 .UNSPECIFIED.);
#330=B_SPLINE_CURVE_WITH_KNOTS('',3,(#13105,#13106,#13107,#13108),
 .UNSPECIFIED.,.F.,.F.,(4,4),(4.51913891174751,8.72381854299666),
 .UNSPECIFIED.);
#331=B_SPLINE_CURVE_WITH_KNOTS('',3,(#13110,#13111,#13112,#13113),
 .UNSPECIFIED.,.F.,.F.,(4,4),(4.46246834806959,8.66714797931881),
 .UNSPECIFIED.);
#332=B_SPLINE_CURVE_WITH_KNOTS('',3,(#13134,#13135,#13136,#13137),
 .UNSPECIFIED.,.F.,.F.,(4,4),(-8.67339028878965,-4.46580127832475),
 .UNSPECIFIED.);
#333=B_SPLINE_CURVE_WITH_KNOTS('',3,(#13156,#13157,#13158,#13159,#13160,
#13161),.UNSPECIFIED.,.F.,.F.,(4,2,4),(-0.607391644691745,-0.303762155877002,
-0.00125172564267001),.UNSPECIFIED.);
#334=B_SPLINE_CURVE_WITH_KNOTS('',3,(#13162,#13163,#13164,#13165,#13166,
#13167,#13168,#13169,#13170,#13171,#13172,#13173,#13174,#13175,#13176,#13177,
#13178,#13179,#13180,#13181,#13182,#13183,#13184,#13185,#13186,#13187,#13188,
#13189),.UNSPECIFIED.,.F.,.F.,(4,3,3,3,3,3,3,3,3,4),(-0.152281539067936,
-0.12854821222061,-0.115190816126163,-0.0912758856104041,-0.0781043161616985,
-0.0652713841318381,-0.0414808619979686,-0.039045740680325,-0.0152551599791835,
0.),.UNSPECIFIED.);
#335=B_SPLINE_CURVE_WITH_KNOTS('',3,(#13191,#13192,#13193,#13194,#13195,
#13196,#13197,#13198,#13199,#13200,#13201,#13202,#13203,#13204,#13205,#13206,
#13207,#13208,#13209,#13210,#13211,#13212,#13213,#13214,#13215,#13216,#13217,
#13218),.UNSPECIFIED.,.F.,.F.,(4,3,3,3,3,3,3,3,3,4),(-0.152284734818265,
-0.128510300097745,-0.115243636037359,-0.0914764658269932,-0.0870316758632336,
-0.078197793898112,-0.0542955901223581,-0.0391042908842167,-0.0153462458625635,
0.),.UNSPECIFIED.);
#336=B_SPLINE_CURVE_WITH_KNOTS('',3,(#13219,#13220,#13221,#13222,#13223,
#13224),.UNSPECIFIED.,.F.,.F.,(4,2,4),(-0.606273164239037,-0.303762187833104,
-0.000133245189939568),.UNSPECIFIED.);
#337=B_SPLINE_CURVE_WITH_KNOTS('',3,(#13241,#13242,#13243,#13244),
 .UNSPECIFIED.,.F.,.F.,(4,4),(-12.1227852464729,-8.92068531110742),
 .UNSPECIFIED.);
#338=B_SPLINE_CURVE_WITH_KNOTS('',3,(#13285,#13286,#13287,#13288),
 .UNSPECIFIED.,.F.,.F.,(4,4),(-4.26560157995882,-1.06350164459338),
 .UNSPECIFIED.);
#339=B_SPLINE_CURVE_WITH_KNOTS('',3,(#13307,#13308,#13309,#13310,#13311,
#13312),.UNSPECIFIED.,.F.,.F.,(4,2,4),(-0.607545900263938,-0.303784727094449,
-0.00134539382494125),.UNSPECIFIED.);
#340=B_SPLINE_CURVE_WITH_KNOTS('',3,(#13314,#13315,#13316,#13317,#13318,
#13319,#13320,#13321,#13322,#13323,#13324,#13325,#13326,#13327,#13328,#13329,
#13330,#13331,#13332,#13333,#13334,#13335,#13336,#13337,#13338,#13339,#13340,
#13341),.UNSPECIFIED.,.F.,.F.,(4,3,3,3,3,3,3,3,3,4),(-0.152214473108837,
-0.128485298747135,-0.115164309990209,-0.0912534321321267,-0.0781163092888813,
-0.0652482412471129,-0.0414606388666645,-0.0390548598067502,-0.0152611452145655,
0.),.UNSPECIFIED.);
#341=B_SPLINE_CURVE_WITH_KNOTS('',3,(#13345,#13346,#13347,#13348,#13349,
#13350,#13351,#13352,#13353,#13354,#13355,#13356,#13357,#13358,#13359,#13360,
#13361,#13362,#13363,#13364,#13365,#13366,#13367,#13368,#13369,#13370,#13371,
#13372),.UNSPECIFIED.,.F.,.F.,(4,3,3,3,3,3,3,3,3,4),(-0.152216110966007,
-0.128438825687404,-0.115191384846861,-0.0914281188167518,-0.0869870566155827,
-0.0781642271790374,-0.0542662950786889,-0.0390848818783988,-0.0153309789665,
0.),.UNSPECIFIED.);
#342=B_SPLINE_CURVE_WITH_KNOTS('',3,(#13373,#13374,#13375,#13376,#13377,
#13378),.UNSPECIFIED.,.F.,.F.,(4,2,4),(-0.606227037063105,-0.303784766192107,
-2.65251918123988E-5),.UNSPECIFIED.);
#343=B_SPLINE_CURVE_WITH_KNOTS('',3,(#13396,#13397,#13398,#13399),
 .UNSPECIFIED.,.F.,.F.,(4,4),(0.0107208554739345,0.617725317592517),
 .UNSPECIFIED.);
#344=B_SPLINE_CURVE_WITH_KNOTS('',3,(#13400,#13401,#13402,#13403),
 .UNSPECIFIED.,.F.,.F.,(4,4),(-12.893479658151,-12.3228618033436),
 .UNSPECIFIED.);
#345=B_SPLINE_CURVE_WITH_KNOTS('',3,(#13426,#13427,#13428,#13429),
 .UNSPECIFIED.,.F.,.F.,(4,4),(12.3251818525939,12.893479658151),
 .UNSPECIFIED.);
#346=B_SPLINE_CURVE_WITH_KNOTS('',3,(#13433,#13434,#13435,#13436),
 .UNSPECIFIED.,.F.,.F.,(4,4),(0.292807233425235,0.861105038472338),
 .UNSPECIFIED.);
#347=B_SPLINE_CURVE_WITH_KNOTS('',3,(#13454,#13455,#13456,#13457),
 .UNSPECIFIED.,.F.,.F.,(4,4),(-0.863425087722636,-0.29280723291527),
 .UNSPECIFIED.);
#348=B_SPLINE_CURVE_WITH_KNOTS('',3,(#13458,#13459,#13460,#13461),
 .UNSPECIFIED.,.F.,.F.,(4,4),(-0.617725317592517,-0.0107208554739345),
 .UNSPECIFIED.);
#349=B_SPLINE_CURVE_WITH_KNOTS('',3,(#13545,#13546,#13547,#13548),
 .UNSPECIFIED.,.F.,.F.,(4,4),(0.00878563933291533,0.615688454110788),
 .UNSPECIFIED.);
#350=B_SPLINE_CURVE_WITH_KNOTS('',3,(#13573,#13574,#13575,#13576),
 .UNSPECIFIED.,.F.,.F.,(4,4),(-0.615688454110787,-0.00878563933291527),
 .UNSPECIFIED.);
#351=B_SPLINE_CURVE_WITH_KNOTS('',3,(#13662,#13663,#13664,#13665),
 .UNSPECIFIED.,.F.,.F.,(4,4),(-9.62771529167128E-17,0.617725317592517),
 .UNSPECIFIED.);
#352=B_SPLINE_CURVE_WITH_KNOTS('',3,(#13666,#13667,#13668,#13669),
 .UNSPECIFIED.,.F.,.F.,(4,4),(-0.617725317592517,-0.000337488966422091),
 .UNSPECIFIED.);
#353=B_SPLINE_CURVE_WITH_KNOTS('',3,(#13705,#13706,#13707,#13708,#13709),
 .UNSPECIFIED.,.F.,.F.,(4,1,4),(-12.893479658151,-5.71764434212835,-0.335767855111383),
 .UNSPECIFIED.);
#354=B_SPLINE_CURVE_WITH_KNOTS('',3,(#13710,#13711,#13712,#13713,#13714),
 .UNSPECIFIED.,.F.,.F.,(4,1,4),(0.335767855111383,5.71764434212835,12.893479658151),
 .UNSPECIFIED.);
#355=B_SPLINE_CURVE_WITH_KNOTS('',3,(#13739,#13740,#13741,#13742),
 .UNSPECIFIED.,.F.,.F.,(4,4),(-0.00171041937131743,0.615688454110788),
 .UNSPECIFIED.);
#356=B_SPLINE_CURVE_WITH_KNOTS('',3,(#13743,#13744,#13745,#13746),
 .UNSPECIFIED.,.F.,.F.,(4,4),(-0.615688454110788,-3.98826847727851E-7),
 .UNSPECIFIED.);
#357=B_SPLINE_CURVE_WITH_KNOTS('',3,(#13771,#13772,#13773,#13774),
 .UNSPECIFIED.,.F.,.F.,(4,4),(3.98826847219577E-7,0.615688454110787),
 .UNSPECIFIED.);
#358=B_SPLINE_CURVE_WITH_KNOTS('',3,(#13775,#13776,#13777,#13778),
 .UNSPECIFIED.,.F.,.F.,(4,4),(-0.615688454110787,0.0017104193713176),
 .UNSPECIFIED.);
#359=B_SPLINE_CURVE_WITH_KNOTS('',3,(#13804,#13805,#13806,#13807,#13808),
 .UNSPECIFIED.,.F.,.F.,(4,1,4),(-12.8505190359549,-7.4686425489379,-0.29280723291527),
 .UNSPECIFIED.);
#360=B_SPLINE_CURVE_WITH_KNOTS('',3,(#13809,#13810,#13811,#13812,#13813),
 .UNSPECIFIED.,.F.,.F.,(4,1,4),(0.292807233425236,7.4686425489379,12.8505190359549),
 .UNSPECIFIED.);
#361=B_SPLINE_CURVE_WITH_KNOTS('',3,(#13834,#13835,#13836,#13837),
 .UNSPECIFIED.,.F.,.F.,(4,4),(0.000337488966421928,0.617725317592517),
 .UNSPECIFIED.);
#362=B_SPLINE_CURVE_WITH_KNOTS('',3,(#13838,#13839,#13840,#13841),
 .UNSPECIFIED.,.F.,.F.,(4,4),(-0.617725317592517,8.06646416329215E-17),
 .UNSPECIFIED.);
#550=SHAPE_REPRESENTATION_RELATIONSHIP('SRR','None',#19670,#560);
#560=ADVANCED_BREP_SHAPE_REPRESENTATION('',(#580),#19613);
#570=STYLED_ITEM('',(#19731),#580);
#580=MANIFOLD_SOLID_BREP('Body1',#7108);
#625=FACE_BOUND('',#1427,.T.);
#626=FACE_BOUND('',#1428,.T.);
#627=FACE_BOUND('',#1429,.T.);
#628=FACE_BOUND('',#1441,.T.);
#629=FACE_BOUND('',#1449,.T.);
#630=FACE_BOUND('',#1460,.T.);
#631=FACE_BOUND('',#1462,.T.);
#632=FACE_BOUND('',#1474,.T.);
#633=FACE_BOUND('',#1483,.T.);
#634=FACE_BOUND('',#1484,.T.);
#635=FACE_BOUND('',#1485,.T.);
#636=FACE_BOUND('',#1534,.T.);
#637=FACE_BOUND('',#1535,.T.);
#638=FACE_BOUND('',#1536,.T.);
#639=FACE_BOUND('',#1537,.T.);
#640=FACE_BOUND('',#1538,.T.);
#641=FACE_BOUND('',#1539,.T.);
#742=PLANE('',#7476);
#743=PLANE('',#7490);
#744=PLANE('',#7491);
#745=PLANE('',#7492);
#746=PLANE('',#7493);
#747=PLANE('',#7494);
#748=PLANE('',#7495);
#749=PLANE('',#7496);
#750=PLANE('',#7498);
#751=PLANE('',#7499);
#752=PLANE('',#7500);
#753=PLANE('',#7501);
#754=PLANE('',#7502);
#755=PLANE('',#7503);
#756=PLANE('',#7504);
#757=PLANE('',#7510);
#758=PLANE('',#7511);
#759=PLANE('',#7512);
#760=PLANE('',#7513);
#761=PLANE('',#7514);
#762=PLANE('',#7515);
#763=PLANE('',#7516);
#764=PLANE('',#7517);
#765=PLANE('',#7519);
#766=PLANE('',#7521);
#767=PLANE('',#7522);
#768=PLANE('',#7523);
#769=PLANE('',#7524);
#770=PLANE('',#7525);
#771=PLANE('',#7526);
#772=PLANE('',#7527);
#773=PLANE('',#7528);
#774=PLANE('',#7529);
#775=PLANE('',#7530);
#776=PLANE('',#7531);
#777=PLANE('',#7535);
#778=PLANE('',#7537);
#779=PLANE('',#7538);
#780=PLANE('',#7539);
#781=PLANE('',#7540);
#782=PLANE('',#7541);
#783=PLANE('',#7542);
#784=PLANE('',#7544);
#785=PLANE('',#7561);
#786=PLANE('',#7580);
#787=PLANE('',#7581);
#788=PLANE('',#7582);
#987=FACE_OUTER_BOUND('',#1426,.T.);
#988=FACE_OUTER_BOUND('',#1430,.T.);
#989=FACE_OUTER_BOUND('',#1431,.T.);
#990=FACE_OUTER_BOUND('',#1432,.T.);
#991=FACE_OUTER_BOUND('',#1433,.T.);
#992=FACE_OUTER_BOUND('',#1434,.T.);
#993=FACE_OUTER_BOUND('',#1435,.T.);
#994=FACE_OUTER_BOUND('',#1436,.T.);
#995=FACE_OUTER_BOUND('',#1437,.T.);
#996=FACE_OUTER_BOUND('',#1438,.T.);
#997=FACE_OUTER_BOUND('',#1439,.T.);
#998=FACE_OUTER_BOUND('',#1440,.T.);
#999=FACE_OUTER_BOUND('',#1442,.T.);
#1000=FACE_OUTER_BOUND('',#1443,.T.);
#1001=FACE_OUTER_BOUND('',#1444,.T.);
#1002=FACE_OUTER_BOUND('',#1445,.T.);
#1003=FACE_OUTER_BOUND('',#1446,.T.);
#1004=FACE_OUTER_BOUND('',#1447,.T.);
#1005=FACE_OUTER_BOUND('',#1448,.T.);
#1006=FACE_OUTER_BOUND('',#1450,.T.);
#1007=FACE_OUTER_BOUND('',#1451,.T.);
#1008=FACE_OUTER_BOUND('',#1452,.T.);
#1009=FACE_OUTER_BOUND('',#1453,.T.);
#1010=FACE_OUTER_BOUND('',#1454,.T.);
#1011=FACE_OUTER_BOUND('',#1455,.T.);
#1012=FACE_OUTER_BOUND('',#1456,.T.);
#1013=FACE_OUTER_BOUND('',#1457,.T.);
#1014=FACE_OUTER_BOUND('',#1458,.T.);
#1015=FACE_OUTER_BOUND('',#1459,.T.);
#1016=FACE_OUTER_BOUND('',#1461,.T.);
#1017=FACE_OUTER_BOUND('',#1463,.T.);
#1018=FACE_OUTER_BOUND('',#1464,.T.);
#1019=FACE_OUTER_BOUND('',#1465,.T.);
#1020=FACE_OUTER_BOUND('',#1466,.T.);
#1021=FACE_OUTER_BOUND('',#1467,.T.);
#1022=FACE_OUTER_BOUND('',#1468,.T.);
#1023=FACE_OUTER_BOUND('',#1469,.T.);
#1024=FACE_OUTER_BOUND('',#1470,.T.);
#1025=FACE_OUTER_BOUND('',#1471,.T.);
#1026=FACE_OUTER_BOUND('',#1472,.T.);
#1027=FACE_OUTER_BOUND('',#1473,.T.);
#1028=FACE_OUTER_BOUND('',#1475,.T.);
#1029=FACE_OUTER_BOUND('',#1476,.T.);
#1030=FACE_OUTER_BOUND('',#1477,.T.);
#1031=FACE_OUTER_BOUND('',#1478,.T.);
#1032=FACE_OUTER_BOUND('',#1479,.T.);
#1033=FACE_OUTER_BOUND('',#1480,.T.);
#1034=FACE_OUTER_BOUND('',#1481,.T.);
#1035=FACE_OUTER_BOUND('',#1482,.T.);
#1036=FACE_OUTER_BOUND('',#1486,.T.);
#1037=FACE_OUTER_BOUND('',#1487,.T.);
#1038=FACE_OUTER_BOUND('',#1488,.T.);
#1039=FACE_OUTER_BOUND('',#1489,.T.);
#1040=FACE_OUTER_BOUND('',#1490,.T.);
#1041=FACE_OUTER_BOUND('',#1491,.T.);
#1042=FACE_OUTER_BOUND('',#1492,.T.);
#1043=FACE_OUTER_BOUND('',#1493,.T.);
#1044=FACE_OUTER_BOUND('',#1494,.T.);
#1045=FACE_OUTER_BOUND('',#1495,.T.);
#1046=FACE_OUTER_BOUND('',#1496,.T.);
#1047=FACE_OUTER_BOUND('',#1497,.T.);
#1048=FACE_OUTER_BOUND('',#1498,.T.);
#1049=FACE_OUTER_BOUND('',#1499,.T.);
#1050=FACE_OUTER_BOUND('',#1500,.T.);
#1051=FACE_OUTER_BOUND('',#1501,.T.);
#1052=FACE_OUTER_BOUND('',#1502,.T.);
#1053=FACE_OUTER_BOUND('',#1503,.T.);
#1054=FACE_OUTER_BOUND('',#1504,.T.);
#1055=FACE_OUTER_BOUND('',#1505,.T.);
#1056=FACE_OUTER_BOUND('',#1506,.T.);
#1057=FACE_OUTER_BOUND('',#1507,.T.);
#1058=FACE_OUTER_BOUND('',#1508,.T.);
#1059=FACE_OUTER_BOUND('',#1509,.T.);
#1060=FACE_OUTER_BOUND('',#1510,.T.);
#1061=FACE_OUTER_BOUND('',#1511,.T.);
#1062=FACE_OUTER_BOUND('',#1512,.T.);
#1063=FACE_OUTER_BOUND('',#1513,.T.);
#1064=FACE_OUTER_BOUND('',#1514,.T.);
#1065=FACE_OUTER_BOUND('',#1515,.T.);
#1066=FACE_OUTER_BOUND('',#1516,.T.);
#1067=FACE_OUTER_BOUND('',#1517,.T.);
#1068=FACE_OUTER_BOUND('',#1518,.T.);
#1069=FACE_OUTER_BOUND('',#1519,.T.);
#1070=FACE_OUTER_BOUND('',#1520,.T.);
#1071=FACE_OUTER_BOUND('',#1521,.T.);
#1072=FACE_OUTER_BOUND('',#1522,.T.);
#1073=FACE_OUTER_BOUND('',#1523,.T.);
#1074=FACE_OUTER_BOUND('',#1524,.T.);
#1075=FACE_OUTER_BOUND('',#1525,.T.);
#1076=FACE_OUTER_BOUND('',#1526,.T.);
#1077=FACE_OUTER_BOUND('',#1527,.T.);
#1078=FACE_OUTER_BOUND('',#1528,.T.);
#1079=FACE_OUTER_BOUND('',#1529,.T.);
#1080=FACE_OUTER_BOUND('',#1530,.T.);
#1081=FACE_OUTER_BOUND('',#1531,.T.);
#1082=FACE_OUTER_BOUND('',#1532,.T.);
#1083=FACE_OUTER_BOUND('',#1533,.T.);
#1084=FACE_OUTER_BOUND('',#1540,.T.);
#1085=FACE_OUTER_BOUND('',#1541,.T.);
#1426=EDGE_LOOP('',(#5342,#5343,#5344,#5345,#5346,#5347,#5348,#5349));
#1427=EDGE_LOOP('',(#5350));
#1428=EDGE_LOOP('',(#5351));
#1429=EDGE_LOOP('',(#5352));
#1430=EDGE_LOOP('',(#5353,#5354,#5355,#5356));
#1431=EDGE_LOOP('',(#5357,#5358,#5359,#5360));
#1432=EDGE_LOOP('',(#5361,#5362,#5363,#5364));
#1433=EDGE_LOOP('',(#5365,#5366,#5367,#5368));
#1434=EDGE_LOOP('',(#5369,#5370,#5371,#5372));
#1435=EDGE_LOOP('',(#5373,#5374,#5375,#5376));
#1436=EDGE_LOOP('',(#5377,#5378,#5379,#5380));
#1437=EDGE_LOOP('',(#5381,#5382,#5383,#5384));
#1438=EDGE_LOOP('',(#5385,#5386,#5387,#5388));
#1439=EDGE_LOOP('',(#5389,#5390,#5391,#5392));
#1440=EDGE_LOOP('',(#5393,#5394,#5395,#5396,#5397,#5398));
#1441=EDGE_LOOP('',(#5399));
#1442=EDGE_LOOP('',(#5400,#5401,#5402,#5403));
#1443=EDGE_LOOP('',(#5404,#5405,#5406,#5407));
#1444=EDGE_LOOP('',(#5408,#5409,#5410,#5411));
#1445=EDGE_LOOP('',(#5412,#5413,#5414,#5415));
#1446=EDGE_LOOP('',(#5416,#5417,#5418,#5419));
#1447=EDGE_LOOP('',(#5420,#5421,#5422,#5423));
#1448=EDGE_LOOP('',(#5424,#5425,#5426,#5427,#5428,#5429));
#1449=EDGE_LOOP('',(#5430));
#1450=EDGE_LOOP('',(#5431,#5432,#5433,#5434));
#1451=EDGE_LOOP('',(#5435,#5436,#5437,#5438));
#1452=EDGE_LOOP('',(#5439,#5440,#5441,#5442));
#1453=EDGE_LOOP('',(#5443,#5444,#5445,#5446));
#1454=EDGE_LOOP('',(#5447,#5448,#5449,#5450));
#1455=EDGE_LOOP('',(#5451,#5452,#5453,#5454));
#1456=EDGE_LOOP('',(#5455,#5456,#5457,#5458));
#1457=EDGE_LOOP('',(#5459,#5460,#5461,#5462));
#1458=EDGE_LOOP('',(#5463,#5464,#5465,#5466));
#1459=EDGE_LOOP('',(#5467));
#1460=EDGE_LOOP('',(#5468));
#1461=EDGE_LOOP('',(#5469));
#1462=EDGE_LOOP('',(#5470));
#1463=EDGE_LOOP('',(#5471,#5472,#5473,#5474));
#1464=EDGE_LOOP('',(#5475,#5476,#5477,#5478));
#1465=EDGE_LOOP('',(#5479,#5480,#5481,#5482));
#1466=EDGE_LOOP('',(#5483,#5484,#5485,#5486));
#1467=EDGE_LOOP('',(#5487,#5488,#5489,#5490));
#1468=EDGE_LOOP('',(#5491,#5492,#5493,#5494,#5495,#5496));
#1469=EDGE_LOOP('',(#5497,#5498,#5499,#5500,#5501,#5502,#5503,#5504,#5505,
#5506));
#1470=EDGE_LOOP('',(#5507,#5508,#5509,#5510,#5511,#5512,#5513,#5514,#5515,
#5516));
#1471=EDGE_LOOP('',(#5517,#5518,#5519,#5520,#5521,#5522,#5523,#5524,#5525,
#5526));
#1472=EDGE_LOOP('',(#5527,#5528,#5529,#5530,#5531,#5532,#5533,#5534));
#1473=EDGE_LOOP('',(#5535,#5536,#5537,#5538,#5539,#5540,#5541,#5542,#5543,
#5544,#5545,#5546,#5547,#5548,#5549,#5550,#5551,#5552,#5553,#5554,#5555,
#5556,#5557,#5558,#5559,#5560,#5561,#5562,#5563,#5564,#5565,#5566,#5567,
#5568,#5569,#5570,#5571,#5572,#5573,#5574,#5575,#5576));
#1474=EDGE_LOOP('',(#5577,#5578,#5579,#5580,#5581,#5582));
#1475=EDGE_LOOP('',(#5583,#5584,#5585,#5586));
#1476=EDGE_LOOP('',(#5587,#5588,#5589,#5590));
#1477=EDGE_LOOP('',(#5591,#5592,#5593,#5594,#5595,#5596));
#1478=EDGE_LOOP('',(#5597,#5598,#5599,#5600));
#1479=EDGE_LOOP('',(#5601,#5602,#5603,#5604));
#1480=EDGE_LOOP('',(#5605,#5606,#5607,#5608));
#1481=EDGE_LOOP('',(#5609,#5610,#5611,#5612));
#1482=EDGE_LOOP('',(#5613,#5614,#5615,#5616));
#1483=EDGE_LOOP('',(#5617));
#1484=EDGE_LOOP('',(#5618));
#1485=EDGE_LOOP('',(#5619));
#1486=EDGE_LOOP('',(#5620,#5621,#5622,#5623));
#1487=EDGE_LOOP('',(#5624,#5625,#5626,#5627));
#1488=EDGE_LOOP('',(#5628,#5629,#5630,#5631));
#1489=EDGE_LOOP('',(#5632,#5633,#5634,#5635));
#1490=EDGE_LOOP('',(#5636,#5637,#5638,#5639,#5640,#5641,#5642,#5643,#5644,
#5645));
#1491=EDGE_LOOP('',(#5646,#5647,#5648,#5649));
#1492=EDGE_LOOP('',(#5650,#5651,#5652,#5653));
#1493=EDGE_LOOP('',(#5654,#5655,#5656,#5657));
#1494=EDGE_LOOP('',(#5658,#5659,#5660,#5661));
#1495=EDGE_LOOP('',(#5662,#5663,#5664,#5665));
#1496=EDGE_LOOP('',(#5666,#5667,#5668,#5669,#5670,#5671,#5672,#5673,#5674,
#5675));
#1497=EDGE_LOOP('',(#5676,#5677,#5678,#5679));
#1498=EDGE_LOOP('',(#5680,#5681,#5682,#5683,#5684,#5685));
#1499=EDGE_LOOP('',(#5686,#5687,#5688,#5689,#5690,#5691));
#1500=EDGE_LOOP('',(#5692,#5693,#5694,#5695));
#1501=EDGE_LOOP('',(#5696,#5697,#5698,#5699,#5700,#5701,#5702,#5703,#5704,
#5705));
#1502=EDGE_LOOP('',(#5706,#5707,#5708,#5709));
#1503=EDGE_LOOP('',(#5710,#5711,#5712,#5713));
#1504=EDGE_LOOP('',(#5714,#5715,#5716,#5717));
#1505=EDGE_LOOP('',(#5718,#5719,#5720,#5721));
#1506=EDGE_LOOP('',(#5722,#5723,#5724,#5725));
#1507=EDGE_LOOP('',(#5726,#5727,#5728));
#1508=EDGE_LOOP('',(#5729,#5730,#5731));
#1509=EDGE_LOOP('',(#5732,#5733,#5734));
#1510=EDGE_LOOP('',(#5735,#5736,#5737,#5738));
#1511=EDGE_LOOP('',(#5739,#5740,#5741,#5742));
#1512=EDGE_LOOP('',(#5743,#5744,#5745));
#1513=EDGE_LOOP('',(#5746,#5747,#5748,#5749));
#1514=EDGE_LOOP('',(#5750,#5751,#5752,#5753));
#1515=EDGE_LOOP('',(#5754,#5755,#5756,#5757));
#1516=EDGE_LOOP('',(#5758,#5759,#5760,#5761));
#1517=EDGE_LOOP('',(#5762,#5763,#5764,#5765));
#1518=EDGE_LOOP('',(#5766,#5767,#5768,#5769));
#1519=EDGE_LOOP('',(#5770,#5771,#5772));
#1520=EDGE_LOOP('',(#5773,#5774,#5775));
#1521=EDGE_LOOP('',(#5776,#5777,#5778));
#1522=EDGE_LOOP('',(#5779,#5780,#5781,#5782));
#1523=EDGE_LOOP('',(#5783,#5784,#5785,#5786));
#1524=EDGE_LOOP('',(#5787,#5788,#5789));
#1525=EDGE_LOOP('',(#5790,#5791,#5792,#5793));
#1526=EDGE_LOOP('',(#5794,#5795,#5796,#5797));
#1527=EDGE_LOOP('',(#5798,#5799,#5800,#5801));
#1528=EDGE_LOOP('',(#5802,#5803,#5804,#5805));
#1529=EDGE_LOOP('',(#5806,#5807,#5808,#5809));
#1530=EDGE_LOOP('',(#5810,#5811,#5812,#5813));
#1531=EDGE_LOOP('',(#5814,#5815,#5816,#5817));
#1532=EDGE_LOOP('',(#5818,#5819,#5820,#5821,#5822,#5823,#5824,#5825));
#1533=EDGE_LOOP('',(#5826,#5827,#5828,#5829));
#1534=EDGE_LOOP('',(#5830,#5831,#5832,#5833,#5834,#5835));
#1535=EDGE_LOOP('',(#5836,#5837,#5838,#5839,#5840,#5841));
#1536=EDGE_LOOP('',(#5842));
#1537=EDGE_LOOP('',(#5843));
#1538=EDGE_LOOP('',(#5844));
#1539=EDGE_LOOP('',(#5845));
#1540=EDGE_LOOP('',(#5846,#5847,#5848,#5849));
#1541=EDGE_LOOP('',(#5850,#5851,#5852,#5853));
#1911=LINE('',#11778,#2370);
#1912=LINE('',#11810,#2371);
#1913=LINE('',#11845,#2372);
#1914=LINE('',#11850,#2373);
#1915=LINE('',#11854,#2374);
#1916=LINE('',#11859,#2375);
#1917=LINE('',#11864,#2376);
#1918=LINE('',#11866,#2377);
#1919=LINE('',#11868,#2378);
#1920=LINE('',#11869,#2379);
#1921=LINE('',#11872,#2380);
#1922=LINE('',#11874,#2381);
#1923=LINE('',#11875,#2382);
#1924=LINE('',#11878,#2383);
#1925=LINE('',#11880,#2384);
#1926=LINE('',#11881,#2385);
#1927=LINE('',#11884,#2386);
#1928=LINE('',#11886,#2387);
#1929=LINE('',#11887,#2388);
#1930=LINE('',#11890,#2389);
#1931=LINE('',#11892,#2390);
#1932=LINE('',#11893,#2391);
#1933=LINE('',#11895,#2392);
#1934=LINE('',#11896,#2393);
#1935=LINE('',#11903,#2394);
#1936=LINE('',#11905,#2395);
#1937=LINE('',#11907,#2396);
#1938=LINE('',#11908,#2397);
#1939=LINE('',#11911,#2398);
#1940=LINE('',#11913,#2399);
#1941=LINE('',#11914,#2400);
#1942=LINE('',#11917,#2401);
#1943=LINE('',#11919,#2402);
#1944=LINE('',#11920,#2403);
#1945=LINE('',#11923,#2404);
#1946=LINE('',#11925,#2405);
#1947=LINE('',#11926,#2406);
#1948=LINE('',#11929,#2407);
#1949=LINE('',#11931,#2408);
#1950=LINE('',#11932,#2409);
#1951=LINE('',#11934,#2410);
#1952=LINE('',#11935,#2411);
#1953=LINE('',#11941,#2412);
#1954=LINE('',#11945,#2413);
#1955=LINE('',#11950,#2414);
#1956=LINE('',#11952,#2415);
#1957=LINE('',#11954,#2416);
#1958=LINE('',#11955,#2417);
#1959=LINE('',#11959,#2418);
#1960=LINE('',#11961,#2419);
#1961=LINE('',#11963,#2420);
#1962=LINE('',#11964,#2421);
#1963=LINE('',#11968,#2422);
#1964=LINE('',#11970,#2423);
#1965=LINE('',#11972,#2424);
#1966=LINE('',#11973,#2425);
#1967=LINE('',#11977,#2426);
#1968=LINE('',#11979,#2427);
#1969=LINE('',#11981,#2428);
#1970=LINE('',#11982,#2429);
#1971=LINE('',#11986,#2430);
#1972=LINE('',#11988,#2431);
#1973=LINE('',#11990,#2432);
#1974=LINE('',#11991,#2433);
#1975=LINE('',#11995,#2434);
#1976=LINE('',#11997,#2435);
#1977=LINE('',#11999,#2436);
#1978=LINE('',#12000,#2437);
#1979=LINE('',#12004,#2438);
#1980=LINE('',#12006,#2439);
#1981=LINE('',#12008,#2440);
#1982=LINE('',#12009,#2441);
#1983=LINE('',#12017,#2442);
#1984=LINE('',#12018,#2443);
#1985=LINE('',#12020,#2444);
#1986=LINE('',#12021,#2445);
#1987=LINE('',#12023,#2446);
#1988=LINE('',#12024,#2447);
#1989=LINE('',#12027,#2448);
#1990=LINE('',#12029,#2449);
#1991=LINE('',#12030,#2450);
#1992=LINE('',#12033,#2451);
#1993=LINE('',#12035,#2452);
#1994=LINE('',#12036,#2453);
#1995=LINE('',#12040,#2454);
#1996=LINE('',#12078,#2455);
#1997=LINE('',#12116,#2456);
#1998=LINE('',#12154,#2457);
#1999=LINE('',#12191,#2458);
#2000=LINE('',#12194,#2459);
#2001=LINE('',#12232,#2460);
#2002=LINE('',#12269,#2461);
#2003=LINE('',#12272,#2462);
#2004=LINE('',#12344,#2463);
#2005=LINE('',#12347,#2464);
#2006=LINE('',#12354,#2465);
#2007=LINE('',#12360,#2466);
#2008=LINE('',#12371,#2467);
#2009=LINE('',#12383,#2468);
#2010=LINE('',#12389,#2469);
#2011=LINE('',#12424,#2470);
#2012=LINE('',#12513,#2471);
#2013=LINE('',#12601,#2472);
#2014=LINE('',#12636,#2473);
#2015=LINE('',#12642,#2474);
#2016=LINE('',#12654,#2475);
#2017=LINE('',#12697,#2476);
#2018=LINE('',#12738,#2477);
#2019=LINE('',#12742,#2478);
#2020=LINE('',#12744,#2479);
#2021=LINE('',#12790,#2480);
#2022=LINE('',#12925,#2481);
#2023=LINE('',#13029,#2482);
#2024=LINE('',#13343,#2483);
#2025=LINE('',#13432,#2484);
#2026=LINE('',#13520,#2485);
#2027=LINE('',#13640,#2486);
#2028=LINE('',#13641,#2487);
#2029=LINE('',#13678,#2488);
#2030=LINE('',#13679,#2489);
#2370=VECTOR('',#8488,1.);
#2371=VECTOR('',#8489,1.);
#2372=VECTOR('',#8500,0.15);
#2373=VECTOR('',#8507,0.15);
#2374=VECTOR('',#8512,0.15);
#2375=VECTOR('',#8517,0.15);
#2376=VECTOR('',#8522,1.);
#2377=VECTOR('',#8523,1.);
#2378=VECTOR('',#8524,1.);
#2379=VECTOR('',#8525,1.);
#2380=VECTOR('',#8528,1.);
#2381=VECTOR('',#8529,1.);
#2382=VECTOR('',#8530,1.);
#2383=VECTOR('',#8533,1.);
#2384=VECTOR('',#8534,1.);
#2385=VECTOR('',#8535,1.);
#2386=VECTOR('',#8538,1.);
#2387=VECTOR('',#8539,1.);
#2388=VECTOR('',#8540,1.);
#2389=VECTOR('',#8543,1.);
#2390=VECTOR('',#8544,1.);
#2391=VECTOR('',#8545,1.);
#2392=VECTOR('',#8548,1.);
#2393=VECTOR('',#8549,1.);
#2394=VECTOR('',#8556,1.);
#2395=VECTOR('',#8557,1.);
#2396=VECTOR('',#8558,1.);
#2397=VECTOR('',#8559,1.);
#2398=VECTOR('',#8562,1.);
#2399=VECTOR('',#8563,1.);
#2400=VECTOR('',#8564,1.);
#2401=VECTOR('',#8567,1.);
#2402=VECTOR('',#8568,1.);
#2403=VECTOR('',#8569,1.);
#2404=VECTOR('',#8572,1.);
#2405=VECTOR('',#8573,1.);
#2406=VECTOR('',#8574,1.);
#2407=VECTOR('',#8577,1.);
#2408=VECTOR('',#8578,1.);
#2409=VECTOR('',#8579,1.);
#2410=VECTOR('',#8582,1.);
#2411=VECTOR('',#8583,1.);
#2412=VECTOR('',#8590,0.17);
#2413=VECTOR('',#8595,0.17);
#2414=VECTOR('',#8600,1.);
#2415=VECTOR('',#8601,1.);
#2416=VECTOR('',#8602,1.);
#2417=VECTOR('',#8603,1.);
#2418=VECTOR('',#8606,1.);
#2419=VECTOR('',#8607,1.);
#2420=VECTOR('',#8608,1.);
#2421=VECTOR('',#8609,1.);
#2422=VECTOR('',#8612,1.);
#2423=VECTOR('',#8613,1.);
#2424=VECTOR('',#8614,1.);
#2425=VECTOR('',#8615,1.);
#2426=VECTOR('',#8618,1.);
#2427=VECTOR('',#8619,1.);
#2428=VECTOR('',#8620,1.);
#2429=VECTOR('',#8621,1.);
#2430=VECTOR('',#8624,1.);
#2431=VECTOR('',#8625,1.);
#2432=VECTOR('',#8626,1.);
#2433=VECTOR('',#8627,1.);
#2434=VECTOR('',#8630,1.);
#2435=VECTOR('',#8631,1.);
#2436=VECTOR('',#8632,1.);
#2437=VECTOR('',#8633,1.);
#2438=VECTOR('',#8636,1.);
#2439=VECTOR('',#8637,1.);
#2440=VECTOR('',#8638,1.);
#2441=VECTOR('',#8639,1.);
#2442=VECTOR('',#8650,1.);
#2443=VECTOR('',#8651,1.);
#2444=VECTOR('',#8654,1.);
#2445=VECTOR('',#8655,1.);
#2446=VECTOR('',#8658,1.);
#2447=VECTOR('',#8659,1.);
#2448=VECTOR('',#8662,1.);
#2449=VECTOR('',#8663,1.);
#2450=VECTOR('',#8664,1.);
#2451=VECTOR('',#8667,1.);
#2452=VECTOR('',#8668,1.);
#2453=VECTOR('',#8669,1.);
#2454=VECTOR('',#8672,1.);
#2455=VECTOR('',#8673,1.);
#2456=VECTOR('',#8676,1.);
#2457=VECTOR('',#8677,1.);
#2458=VECTOR('',#8678,1.);
#2459=VECTOR('',#8681,1.);
#2460=VECTOR('',#8682,1.);
#2461=VECTOR('',#8683,1.);
#2462=VECTOR('',#8686,1.);
#2463=VECTOR('',#8687,1.);
#2464=VECTOR('',#8690,1.);
#2465=VECTOR('',#8691,1.);
#2466=VECTOR('',#8692,1.);
#2467=VECTOR('',#8695,1.);
#2468=VECTOR('',#8696,1.);
#2469=VECTOR('',#8697,1.);
#2470=VECTOR('',#8698,1.);
#2471=VECTOR('',#8699,1.);
#2472=VECTOR('',#8700,1.);
#2473=VECTOR('',#8701,1.);
#2474=VECTOR('',#8702,1.);
#2475=VECTOR('',#8703,1.);
#2476=VECTOR('',#8704,1.);
#2477=VECTOR('',#8705,1.);
#2478=VECTOR('',#8710,0.4);
#2479=VECTOR('',#8713,0.4);
#2480=VECTOR('',#8716,1.);
#2481=VECTOR('',#8723,1.);
#2482=VECTOR('',#8726,1.);
#2483=VECTOR('',#8733,1.);
#2484=VECTOR('',#8738,1.);
#2485=VECTOR('',#8771,1.);
#2486=VECTOR('',#8800,1.);
#2487=VECTOR('',#8801,1.);
#2488=VECTOR('',#8812,1.);
#2489=VECTOR('',#8813,1.);
#2726=CIRCLE('',#7477,0.15);
#2727=CIRCLE('',#7478,0.15);
#2728=CIRCLE('',#7479,0.4);
#2729=CIRCLE('',#7481,0.15);
#2730=CIRCLE('',#7482,0.15);
#2731=CIRCLE('',#7484,0.15);
#2732=CIRCLE('',#7486,0.15);
#2733=CIRCLE('',#7488,0.15);
#2734=CIRCLE('',#7489,0.15);
#2735=CIRCLE('',#7497,0.17);
#2736=CIRCLE('',#7505,0.17);
#2737=CIRCLE('',#7507,0.17);
#2738=CIRCLE('',#7509,0.17);
#2739=CIRCLE('',#7518,0.4);
#2740=CIRCLE('',#7520,0.4);
#2741=CIRCLE('',#7533,0.4);
#2742=CIRCLE('',#7536,0.1);
#2743=CIRCLE('',#7543,0.0999999999999999);
#2744=CIRCLE('',#7545,0.0999999999999999);
#2745=CIRCLE('',#7547,0.0999999999999999);
#2746=CIRCLE('',#7548,0.1);
#2747=CIRCLE('',#7550,0.0999999999999998);
#2748=CIRCLE('',#7551,0.0999999999999998);
#2749=CIRCLE('',#7552,0.0999999999999997);
#2750=CIRCLE('',#7554,0.0999999999999998);
#2751=CIRCLE('',#7555,0.0999999999999998);
#2752=CIRCLE('',#7558,0.0999999999999999);
#2753=CIRCLE('',#7559,0.1);
#2754=CIRCLE('',#7563,0.3);
#2755=CIRCLE('',#7564,0.3);
#2756=CIRCLE('',#7565,0.3);
#2757=CIRCLE('',#7567,0.3);
#2758=CIRCLE('',#7568,0.3);
#2759=CIRCLE('',#7569,0.3);
#2760=CIRCLE('',#7571,0.3);
#2761=CIRCLE('',#7572,0.3);
#2762=CIRCLE('',#7573,0.3);
#2763=CIRCLE('',#7576,0.3);
#2764=CIRCLE('',#7577,0.3);
#2765=CIRCLE('',#7578,0.3);
#3081=VERTEX_POINT('',#11771);
#3082=VERTEX_POINT('',#11772);
#3083=VERTEX_POINT('',#11777);
#3084=VERTEX_POINT('',#11779);
#3085=VERTEX_POINT('',#11784);
#3086=VERTEX_POINT('',#11804);
#3087=VERTEX_POINT('',#11809);
#3088=VERTEX_POINT('',#11811);
#3089=VERTEX_POINT('',#11835);
#3090=VERTEX_POINT('',#11837);
#3091=VERTEX_POINT('',#11839);
#3092=VERTEX_POINT('',#11842);
#3093=VERTEX_POINT('',#11844);
#3094=VERTEX_POINT('',#11848);
#3095=VERTEX_POINT('',#11852);
#3096=VERTEX_POINT('',#11856);
#3097=VERTEX_POINT('',#11858);
#3098=VERTEX_POINT('',#11862);
#3099=VERTEX_POINT('',#11863);
#3100=VERTEX_POINT('',#11865);
#3101=VERTEX_POINT('',#11867);
#3102=VERTEX_POINT('',#11871);
#3103=VERTEX_POINT('',#11873);
#3104=VERTEX_POINT('',#11877);
#3105=VERTEX_POINT('',#11879);
#3106=VERTEX_POINT('',#11883);
#3107=VERTEX_POINT('',#11885);
#3108=VERTEX_POINT('',#11889);
#3109=VERTEX_POINT('',#11891);
#3110=VERTEX_POINT('',#11898);
#3111=VERTEX_POINT('',#11901);
#3112=VERTEX_POINT('',#11902);
#3113=VERTEX_POINT('',#11904);
#3114=VERTEX_POINT('',#11906);
#3115=VERTEX_POINT('',#11910);
#3116=VERTEX_POINT('',#11912);
#3117=VERTEX_POINT('',#11916);
#3118=VERTEX_POINT('',#11918);
#3119=VERTEX_POINT('',#11922);
#3120=VERTEX_POINT('',#11924);
#3121=VERTEX_POINT('',#11928);
#3122=VERTEX_POINT('',#11930);
#3123=VERTEX_POINT('',#11937);
#3124=VERTEX_POINT('',#11940);
#3125=VERTEX_POINT('',#11944);
#3126=VERTEX_POINT('',#11948);
#3127=VERTEX_POINT('',#11949);
#3128=VERTEX_POINT('',#11951);
#3129=VERTEX_POINT('',#11953);
#3130=VERTEX_POINT('',#11957);
#3131=VERTEX_POINT('',#11958);
#3132=VERTEX_POINT('',#11960);
#3133=VERTEX_POINT('',#11962);
#3134=VERTEX_POINT('',#11966);
#3135=VERTEX_POINT('',#11967);
#3136=VERTEX_POINT('',#11969);
#3137=VERTEX_POINT('',#11971);
#3138=VERTEX_POINT('',#11975);
#3139=VERTEX_POINT('',#11976);
#3140=VERTEX_POINT('',#11978);
#3141=VERTEX_POINT('',#11980);
#3142=VERTEX_POINT('',#11984);
#3143=VERTEX_POINT('',#11985);
#3144=VERTEX_POINT('',#11987);
#3145=VERTEX_POINT('',#11989);
#3146=VERTEX_POINT('',#11993);
#3147=VERTEX_POINT('',#11994);
#3148=VERTEX_POINT('',#11996);
#3149=VERTEX_POINT('',#11998);
#3150=VERTEX_POINT('',#12002);
#3151=VERTEX_POINT('',#12003);
#3152=VERTEX_POINT('',#12005);
#3153=VERTEX_POINT('',#12007);
#3154=VERTEX_POINT('',#12011);
#3155=VERTEX_POINT('',#12014);
#3156=VERTEX_POINT('',#12026);
#3157=VERTEX_POINT('',#12028);
#3158=VERTEX_POINT('',#12032);
#3159=VERTEX_POINT('',#12034);
#3160=VERTEX_POINT('',#12038);
#3161=VERTEX_POINT('',#12039);
#3162=VERTEX_POINT('',#12041);
#3163=VERTEX_POINT('',#12048);
#3164=VERTEX_POINT('',#12077);
#3165=VERTEX_POINT('',#12079);
#3166=VERTEX_POINT('',#12115);
#3167=VERTEX_POINT('',#12117);
#3168=VERTEX_POINT('',#12124);
#3169=VERTEX_POINT('',#12153);
#3170=VERTEX_POINT('',#12155);
#3171=VERTEX_POINT('',#12184);
#3172=VERTEX_POINT('',#12193);
#3173=VERTEX_POINT('',#12195);
#3174=VERTEX_POINT('',#12202);
#3175=VERTEX_POINT('',#12231);
#3176=VERTEX_POINT('',#12233);
#3177=VERTEX_POINT('',#12262);
#3178=VERTEX_POINT('',#12271);
#3179=VERTEX_POINT('',#12273);
#3180=VERTEX_POINT('',#12308);
#3181=VERTEX_POINT('',#12337);
#3182=VERTEX_POINT('',#12346);
#3183=VERTEX_POINT('',#12348);
#3184=VERTEX_POINT('',#12353);
#3185=VERTEX_POINT('',#12355);
#3186=VERTEX_POINT('',#12370);
#3187=VERTEX_POINT('',#12382);
#3188=VERTEX_POINT('',#12388);
#3189=VERTEX_POINT('',#12390);
#3190=VERTEX_POINT('',#12423);
#3191=VERTEX_POINT('',#12425);
#3192=VERTEX_POINT('',#12463);
#3193=VERTEX_POINT('',#12468);
#3194=VERTEX_POINT('',#12512);
#3195=VERTEX_POINT('',#12514);
#3196=VERTEX_POINT('',#12558);
#3197=VERTEX_POINT('',#12563);
#3198=VERTEX_POINT('',#12602);
#3199=VERTEX_POINT('',#12631);
#3200=VERTEX_POINT('',#12637);
#3201=VERTEX_POINT('',#12643);
#3202=VERTEX_POINT('',#12655);
#3203=VERTEX_POINT('',#12656);
#3204=VERTEX_POINT('',#12661);
#3205=VERTEX_POINT('',#12696);
#3206=VERTEX_POINT('',#12698);
#3207=VERTEX_POINT('',#12733);
#3208=VERTEX_POINT('',#12740);
#3209=VERTEX_POINT('',#12746);
#3210=VERTEX_POINT('',#12753);
#3211=VERTEX_POINT('',#12760);
#3212=VERTEX_POINT('',#12789);
#3213=VERTEX_POINT('',#12855);
#3214=VERTEX_POINT('',#12908);
#3215=VERTEX_POINT('',#12920);
#3216=VERTEX_POINT('',#12982);
#3217=VERTEX_POINT('',#12992);
#3218=VERTEX_POINT('',#12999);
#3219=VERTEX_POINT('',#13028);
#3220=VERTEX_POINT('',#13030);
#3221=VERTEX_POINT('',#13155);
#3222=VERTEX_POINT('',#13190);
#3223=VERTEX_POINT('',#13306);
#3224=VERTEX_POINT('',#13313);
#3225=VERTEX_POINT('',#13342);
#3226=VERTEX_POINT('',#13344);
#3227=VERTEX_POINT('',#13395);
#3228=VERTEX_POINT('',#13424);
#3229=VERTEX_POINT('',#13431);
#3230=VERTEX_POINT('',#13453);
#3231=VERTEX_POINT('',#13488);
#3232=VERTEX_POINT('',#13516);
#3233=VERTEX_POINT('',#13619);
#3234=VERTEX_POINT('',#13620);
#3235=VERTEX_POINT('',#13622);
#3236=VERTEX_POINT('',#13626);
#3237=VERTEX_POINT('',#13627);
#3238=VERTEX_POINT('',#13629);
#3239=VERTEX_POINT('',#13633);
#3240=VERTEX_POINT('',#13634);
#3241=VERTEX_POINT('',#13636);
#3242=VERTEX_POINT('',#13671);
#3243=VERTEX_POINT('',#13672);
#3244=VERTEX_POINT('',#13674);
#3896=EDGE_CURVE('',#3081,#3082,#267,.T.);
#3897=EDGE_CURVE('',#3082,#3083,#1911,.T.);
#3898=EDGE_CURVE('',#3083,#3084,#268,.T.);
#3899=EDGE_CURVE('',#3085,#3084,#269,.T.);
#3900=EDGE_CURVE('',#3085,#3086,#270,.T.);
#3901=EDGE_CURVE('',#3086,#3087,#1912,.T.);
#3902=EDGE_CURVE('',#3087,#3088,#271,.T.);
#3903=EDGE_CURVE('',#3081,#3088,#272,.T.);
#3904=EDGE_CURVE('',#3089,#3089,#2726,.T.);
#3905=EDGE_CURVE('',#3090,#3090,#2727,.T.);
#3906=EDGE_CURVE('',#3091,#3091,#2728,.T.);
#3907=EDGE_CURVE('',#3092,#3092,#2729,.T.);
#3908=EDGE_CURVE('',#3092,#3093,#1913,.T.);
#3909=EDGE_CURVE('',#3093,#3093,#2730,.T.);
#3910=EDGE_CURVE('',#3094,#3094,#2731,.T.);
#3911=EDGE_CURVE('',#3094,#3090,#1914,.T.);
#3912=EDGE_CURVE('',#3095,#3095,#2732,.T.);
#3913=EDGE_CURVE('',#3095,#3089,#1915,.T.);
#3914=EDGE_CURVE('',#3096,#3096,#2733,.T.);
#3915=EDGE_CURVE('',#3096,#3097,#1916,.T.);
#3916=EDGE_CURVE('',#3097,#3097,#2734,.T.);
#3917=EDGE_CURVE('',#3098,#3099,#1917,.T.);
#3918=EDGE_CURVE('',#3098,#3100,#1918,.T.);
#3919=EDGE_CURVE('',#3100,#3101,#1919,.T.);
#3920=EDGE_CURVE('',#3099,#3101,#1920,.T.);
#3921=EDGE_CURVE('',#3102,#3098,#1921,.T.);
#3922=EDGE_CURVE('',#3102,#3103,#1922,.T.);
#3923=EDGE_CURVE('',#3103,#3100,#1923,.T.);
#3924=EDGE_CURVE('',#3104,#3102,#1924,.T.);
#3925=EDGE_CURVE('',#3104,#3105,#1925,.T.);
#3926=EDGE_CURVE('',#3105,#3103,#1926,.T.);
#3927=EDGE_CURVE('',#3106,#3104,#1927,.T.);
#3928=EDGE_CURVE('',#3106,#3107,#1928,.T.);
#3929=EDGE_CURVE('',#3107,#3105,#1929,.T.);
#3930=EDGE_CURVE('',#3108,#3106,#1930,.T.);
#3931=EDGE_CURVE('',#3108,#3109,#1931,.T.);
#3932=EDGE_CURVE('',#3109,#3107,#1932,.T.);
#3933=EDGE_CURVE('',#3099,#3108,#1933,.T.);
#3934=EDGE_CURVE('',#3101,#3109,#1934,.T.);
#3935=EDGE_CURVE('',#3110,#3110,#2735,.T.);
#3936=EDGE_CURVE('',#3111,#3112,#1935,.T.);
#3937=EDGE_CURVE('',#3111,#3113,#1936,.T.);
#3938=EDGE_CURVE('',#3113,#3114,#1937,.T.);
#3939=EDGE_CURVE('',#3112,#3114,#1938,.T.);
#3940=EDGE_CURVE('',#3115,#3111,#1939,.T.);
#3941=EDGE_CURVE('',#3115,#3116,#1940,.T.);
#3942=EDGE_CURVE('',#3116,#3113,#1941,.T.);
#3943=EDGE_CURVE('',#3117,#3115,#1942,.T.);
#3944=EDGE_CURVE('',#3117,#3118,#1943,.T.);
#3945=EDGE_CURVE('',#3118,#3116,#1944,.T.);
#3946=EDGE_CURVE('',#3119,#3117,#1945,.T.);
#3947=EDGE_CURVE('',#3119,#3120,#1946,.T.);
#3948=EDGE_CURVE('',#3120,#3118,#1947,.T.);
#3949=EDGE_CURVE('',#3121,#3119,#1948,.T.);
#3950=EDGE_CURVE('',#3121,#3122,#1949,.T.);
#3951=EDGE_CURVE('',#3122,#3120,#1950,.T.);
#3952=EDGE_CURVE('',#3112,#3121,#1951,.T.);
#3953=EDGE_CURVE('',#3114,#3122,#1952,.T.);
#3954=EDGE_CURVE('',#3123,#3123,#2736,.T.);
#3955=EDGE_CURVE('',#3123,#3124,#1953,.T.);
#3956=EDGE_CURVE('',#3124,#3124,#2737,.T.);
#3957=EDGE_CURVE('',#3110,#3125,#1954,.T.);
#3958=EDGE_CURVE('',#3125,#3125,#2738,.T.);
#3959=EDGE_CURVE('',#3126,#3127,#1955,.T.);
#3960=EDGE_CURVE('',#3128,#3126,#1956,.T.);
#3961=EDGE_CURVE('',#3129,#3128,#1957,.T.);
#3962=EDGE_CURVE('',#3129,#3127,#1958,.T.);
#3963=EDGE_CURVE('',#3130,#3131,#1959,.T.);
#3964=EDGE_CURVE('',#3130,#3132,#1960,.T.);
#3965=EDGE_CURVE('',#3133,#3132,#1961,.T.);
#3966=EDGE_CURVE('',#3131,#3133,#1962,.T.);
#3967=EDGE_CURVE('',#3134,#3135,#1963,.T.);
#3968=EDGE_CURVE('',#3134,#3136,#1964,.T.);
#3969=EDGE_CURVE('',#3137,#3136,#1965,.T.);
#3970=EDGE_CURVE('',#3135,#3137,#1966,.T.);
#3971=EDGE_CURVE('',#3138,#3139,#1967,.T.);
#3972=EDGE_CURVE('',#3138,#3140,#1968,.T.);
#3973=EDGE_CURVE('',#3141,#3140,#1969,.T.);
#3974=EDGE_CURVE('',#3139,#3141,#1970,.T.);
#3975=EDGE_CURVE('',#3142,#3143,#1971,.T.);
#3976=EDGE_CURVE('',#3142,#3144,#1972,.T.);
#3977=EDGE_CURVE('',#3145,#3144,#1973,.T.);
#3978=EDGE_CURVE('',#3143,#3145,#1974,.T.);
#3979=EDGE_CURVE('',#3146,#3147,#1975,.T.);
#3980=EDGE_CURVE('',#3148,#3146,#1976,.T.);
#3981=EDGE_CURVE('',#3149,#3148,#1977,.T.);
#3982=EDGE_CURVE('',#3149,#3147,#1978,.T.);
#3983=EDGE_CURVE('',#3150,#3151,#1979,.T.);
#3984=EDGE_CURVE('',#3152,#3150,#1980,.T.);
#3985=EDGE_CURVE('',#3153,#3152,#1981,.T.);
#3986=EDGE_CURVE('',#3153,#3151,#1982,.T.);
#3987=EDGE_CURVE('',#3154,#3154,#2739,.T.);
#3988=EDGE_CURVE('',#3155,#3155,#2740,.T.);
#3989=EDGE_CURVE('',#3127,#3142,#1983,.T.);
#3990=EDGE_CURVE('',#3144,#3129,#1984,.T.);
#3991=EDGE_CURVE('',#3147,#3130,#1985,.T.);
#3992=EDGE_CURVE('',#3132,#3149,#1986,.T.);
#3993=EDGE_CURVE('',#3151,#3134,#1987,.T.);
#3994=EDGE_CURVE('',#3136,#3153,#1988,.T.);
#3995=EDGE_CURVE('',#3156,#3138,#1989,.T.);
#3996=EDGE_CURVE('',#3157,#3156,#1990,.T.);
#3997=EDGE_CURVE('',#3140,#3157,#1991,.T.);
#3998=EDGE_CURVE('',#3158,#3156,#1992,.T.);
#3999=EDGE_CURVE('',#3159,#3158,#1993,.T.);
#4000=EDGE_CURVE('',#3157,#3159,#1994,.T.);
#4001=EDGE_CURVE('',#3160,#3161,#1995,.T.);
#4002=EDGE_CURVE('',#3162,#3161,#273,.T.);
#4003=EDGE_CURVE('',#3163,#3162,#274,.T.);
#4004=EDGE_CURVE('',#3164,#3163,#1996,.T.);
#4005=EDGE_CURVE('',#3165,#3164,#275,.T.);
#4006=EDGE_CURVE('',#3160,#3165,#276,.T.);
#4007=EDGE_CURVE('',#3159,#3166,#1997,.T.);
#4008=EDGE_CURVE('',#3167,#3166,#277,.T.);
#4009=EDGE_CURVE('',#3168,#3167,#278,.T.);
#4010=EDGE_CURVE('',#3169,#3168,#1998,.T.);
#4011=EDGE_CURVE('',#3170,#3169,#279,.T.);
#4012=EDGE_CURVE('',#3171,#3170,#280,.T.);
#4013=EDGE_CURVE('',#3171,#3141,#1999,.T.);
#4014=EDGE_CURVE('',#3152,#3172,#2000,.T.);
#4015=EDGE_CURVE('',#3173,#3172,#281,.T.);
#4016=EDGE_CURVE('',#3174,#3173,#282,.T.);
#4017=EDGE_CURVE('',#3175,#3174,#2001,.T.);
#4018=EDGE_CURVE('',#3176,#3175,#283,.T.);
#4019=EDGE_CURVE('',#3177,#3176,#284,.T.);
#4020=EDGE_CURVE('',#3177,#3137,#2002,.T.);
#4021=EDGE_CURVE('',#3148,#3178,#2003,.T.);
#4022=EDGE_CURVE('',#3179,#3178,#285,.T.);
#4023=EDGE_CURVE('',#3087,#3179,#286,.T.);
#4024=EDGE_CURVE('',#3180,#3086,#287,.T.);
#4025=EDGE_CURVE('',#3181,#3180,#288,.T.);
#4026=EDGE_CURVE('',#3181,#3133,#2004,.T.);
#4027=EDGE_CURVE('',#3182,#3143,#2005,.T.);
#4028=EDGE_CURVE('',#3182,#3183,#289,.T.);
#4029=EDGE_CURVE('',#3183,#3184,#2006,.T.);
#4030=EDGE_CURVE('',#3184,#3185,#290,.T.);
#4031=EDGE_CURVE('',#3126,#3185,#2007,.T.);
#4032=EDGE_CURVE('',#3171,#3161,#291,.T.);
#4033=EDGE_CURVE('',#3160,#3166,#292,.T.);
#4034=EDGE_CURVE('',#3186,#3158,#2008,.T.);
#4035=EDGE_CURVE('',#3186,#3172,#293,.T.);
#4036=EDGE_CURVE('',#3187,#3150,#2009,.T.);
#4037=EDGE_CURVE('',#3187,#3178,#294,.T.);
#4038=EDGE_CURVE('',#3188,#3146,#2010,.T.);
#4039=EDGE_CURVE('',#3188,#3189,#295,.T.);
#4040=EDGE_CURVE('',#3189,#3182,#296,.T.);
#4041=EDGE_CURVE('',#3145,#3190,#2011,.T.);
#4042=EDGE_CURVE('',#3191,#3190,#297,.T.);
#4043=EDGE_CURVE('',#3191,#3192,#298,.T.);
#4044=EDGE_CURVE('',#3193,#3192,#299,.T.);
#4045=EDGE_CURVE('',#3193,#3194,#2012,.T.);
#4046=EDGE_CURVE('',#3195,#3194,#300,.T.);
#4047=EDGE_CURVE('',#3195,#3196,#301,.T.);
#4048=EDGE_CURVE('',#3197,#3196,#302,.T.);
#4049=EDGE_CURVE('',#3197,#3128,#2013,.T.);
#4050=EDGE_CURVE('',#3185,#3198,#303,.T.);
#4051=EDGE_CURVE('',#3198,#3199,#304,.T.);
#4052=EDGE_CURVE('',#3131,#3199,#2014,.T.);
#4053=EDGE_CURVE('',#3181,#3200,#305,.T.);
#4054=EDGE_CURVE('',#3135,#3200,#2015,.T.);
#4055=EDGE_CURVE('',#3177,#3201,#306,.T.);
#4056=EDGE_CURVE('',#3139,#3201,#2016,.T.);
#4057=EDGE_CURVE('',#3202,#3203,#307,.T.);
#4058=EDGE_CURVE('',#3203,#3204,#308,.T.);
#4059=EDGE_CURVE('',#3204,#3205,#2017,.T.);
#4060=EDGE_CURVE('',#3205,#3206,#309,.T.);
#4061=EDGE_CURVE('',#3206,#3207,#310,.T.);
#4062=EDGE_CURVE('',#3202,#3207,#2018,.T.);
#4063=EDGE_CURVE('',#3208,#3208,#2741,.T.);
#4064=EDGE_CURVE('',#3208,#3155,#2019,.T.);
#4065=EDGE_CURVE('',#3091,#3154,#2020,.T.);
#4066=EDGE_CURVE('',#3202,#3209,#311,.T.);
#4067=EDGE_CURVE('',#3210,#3207,#312,.T.);
#4068=EDGE_CURVE('',#3211,#3210,#313,.T.);
#4069=EDGE_CURVE('',#3212,#3211,#2021,.T.);
#4070=EDGE_CURVE('',#3209,#3212,#314,.T.);
#4071=EDGE_CURVE('',#3170,#3162,#315,.T.);
#4072=EDGE_CURVE('',#3209,#3213,#316,.T.);
#4073=EDGE_CURVE('',#3213,#3203,#317,.T.);
#4074=EDGE_CURVE('',#3163,#3169,#318,.T.);
#4075=EDGE_CURVE('',#3214,#3212,#319,.T.);
#4076=EDGE_CURVE('',#3213,#3214,#2742,.F.);
#4077=EDGE_CURVE('',#3168,#3164,#320,.T.);
#4078=EDGE_CURVE('',#3211,#3215,#321,.T.);
#4079=EDGE_CURVE('',#3215,#3214,#2022,.T.);
#4080=EDGE_CURVE('',#3165,#3167,#322,.T.);
#4081=EDGE_CURVE('',#3206,#3216,#323,.T.);
#4082=EDGE_CURVE('',#3216,#3210,#324,.T.);
#4083=EDGE_CURVE('',#3217,#3201,#325,.T.);
#4084=EDGE_CURVE('',#3218,#3217,#326,.T.);
#4085=EDGE_CURVE('',#3219,#3218,#2023,.T.);
#4086=EDGE_CURVE('',#3220,#3219,#327,.T.);
#4087=EDGE_CURVE('',#3186,#3220,#328,.T.);
#4088=EDGE_CURVE('',#3176,#3217,#329,.T.);
#4089=EDGE_CURVE('',#3218,#3175,#330,.T.);
#4090=EDGE_CURVE('',#3174,#3219,#331,.T.);
#4091=EDGE_CURVE('',#3220,#3173,#332,.T.);
#4092=EDGE_CURVE('',#3221,#3200,#333,.T.);
#4093=EDGE_CURVE('',#3083,#3221,#334,.T.);
#4094=EDGE_CURVE('',#3222,#3082,#335,.T.);
#4095=EDGE_CURVE('',#3187,#3222,#336,.T.);
#4096=EDGE_CURVE('',#3180,#3221,#337,.T.);
#4097=EDGE_CURVE('',#3222,#3179,#338,.T.);
#4098=EDGE_CURVE('',#3223,#3199,#339,.T.);
#4099=EDGE_CURVE('',#3224,#3223,#340,.T.);
#4100=EDGE_CURVE('',#3225,#3224,#2024,.T.);
#4101=EDGE_CURVE('',#3226,#3225,#341,.T.);
#4102=EDGE_CURVE('',#3188,#3226,#342,.T.);
#4103=EDGE_CURVE('',#3198,#3227,#343,.T.);
#4104=EDGE_CURVE('',#3227,#3223,#344,.T.);
#4105=EDGE_CURVE('',#3228,#3227,#2743,.F.);
#4106=EDGE_CURVE('',#3224,#3228,#345,.T.);
#4107=EDGE_CURVE('',#3228,#3229,#2025,.T.);
#4108=EDGE_CURVE('',#3229,#3225,#346,.T.);
#4109=EDGE_CURVE('',#3226,#3230,#347,.T.);
#4110=EDGE_CURVE('',#3230,#3189,#348,.T.);
#4111=EDGE_CURVE('',#3230,#3229,#2744,.F.);
#4112=EDGE_CURVE('',#3229,#3183,#2745,.F.);
#4113=EDGE_CURVE('',#3183,#3230,#2746,.F.);
#4114=EDGE_CURVE('',#3215,#3216,#2747,.F.);
#4115=EDGE_CURVE('',#3216,#3231,#2748,.F.);
#4116=EDGE_CURVE('',#3231,#3215,#2749,.F.);
#4117=EDGE_CURVE('',#3227,#3184,#2750,.F.);
#4118=EDGE_CURVE('',#3184,#3228,#2751,.F.);
#4119=EDGE_CURVE('',#3232,#3213,#2752,.F.);
#4120=EDGE_CURVE('',#3214,#3232,#2753,.F.);
#4121=EDGE_CURVE('',#3232,#3231,#2026,.T.);
#4122=EDGE_CURVE('',#3204,#3232,#349,.T.);
#4123=EDGE_CURVE('',#3231,#3205,#350,.T.);
#4124=EDGE_CURVE('',#3233,#3234,#2754,.F.);
#4125=EDGE_CURVE('',#3235,#3233,#2755,.F.);
#4126=EDGE_CURVE('',#3234,#3235,#2756,.F.);
#4127=EDGE_CURVE('',#3236,#3237,#2757,.F.);
#4128=EDGE_CURVE('',#3238,#3236,#2758,.F.);
#4129=EDGE_CURVE('',#3237,#3238,#2759,.F.);
#4130=EDGE_CURVE('',#3239,#3240,#2760,.F.);
#4131=EDGE_CURVE('',#3241,#3239,#2761,.F.);
#4132=EDGE_CURVE('',#3240,#3241,#2762,.F.);
#4133=EDGE_CURVE('',#3234,#3241,#2027,.T.);
#4134=EDGE_CURVE('',#3239,#3233,#2028,.T.);
#4135=EDGE_CURVE('',#3196,#3240,#351,.T.);
#4136=EDGE_CURVE('',#3241,#3197,#352,.T.);
#4137=EDGE_CURVE('',#3242,#3243,#2763,.F.);
#4138=EDGE_CURVE('',#3244,#3242,#2764,.F.);
#4139=EDGE_CURVE('',#3243,#3244,#2765,.F.);
#4140=EDGE_CURVE('',#3242,#3238,#2029,.T.);
#4141=EDGE_CURVE('',#3236,#3244,#2030,.T.);
#4142=EDGE_CURVE('',#3240,#3243,#353,.T.);
#4143=EDGE_CURVE('',#3244,#3239,#354,.T.);
#4144=EDGE_CURVE('',#3194,#3242,#355,.T.);
#4145=EDGE_CURVE('',#3243,#3195,#356,.T.);
#4146=EDGE_CURVE('',#3192,#3237,#357,.T.);
#4147=EDGE_CURVE('',#3238,#3193,#358,.T.);
#4148=EDGE_CURVE('',#3237,#3235,#359,.T.);
#4149=EDGE_CURVE('',#3233,#3236,#360,.T.);
#4150=EDGE_CURVE('',#3190,#3234,#361,.T.);
#4151=EDGE_CURVE('',#3235,#3191,#362,.T.);
#5342=ORIENTED_EDGE('',*,*,#3896,.T.);
#5343=ORIENTED_EDGE('',*,*,#3897,.T.);
#5344=ORIENTED_EDGE('',*,*,#3898,.T.);
#5345=ORIENTED_EDGE('',*,*,#3899,.F.);
#5346=ORIENTED_EDGE('',*,*,#3900,.T.);
#5347=ORIENTED_EDGE('',*,*,#3901,.T.);
#5348=ORIENTED_EDGE('',*,*,#3902,.T.);
#5349=ORIENTED_EDGE('',*,*,#3903,.F.);
#5350=ORIENTED_EDGE('',*,*,#3904,.T.);
#5351=ORIENTED_EDGE('',*,*,#3905,.T.);
#5352=ORIENTED_EDGE('',*,*,#3906,.T.);
#5353=ORIENTED_EDGE('',*,*,#3907,.F.);
#5354=ORIENTED_EDGE('',*,*,#3908,.T.);
#5355=ORIENTED_EDGE('',*,*,#3909,.F.);
#5356=ORIENTED_EDGE('',*,*,#3908,.F.);
#5357=ORIENTED_EDGE('',*,*,#3910,.F.);
#5358=ORIENTED_EDGE('',*,*,#3911,.T.);
#5359=ORIENTED_EDGE('',*,*,#3905,.F.);
#5360=ORIENTED_EDGE('',*,*,#3911,.F.);
#5361=ORIENTED_EDGE('',*,*,#3912,.F.);
#5362=ORIENTED_EDGE('',*,*,#3913,.T.);
#5363=ORIENTED_EDGE('',*,*,#3904,.F.);
#5364=ORIENTED_EDGE('',*,*,#3913,.F.);
#5365=ORIENTED_EDGE('',*,*,#3914,.F.);
#5366=ORIENTED_EDGE('',*,*,#3915,.T.);
#5367=ORIENTED_EDGE('',*,*,#3916,.F.);
#5368=ORIENTED_EDGE('',*,*,#3915,.F.);
#5369=ORIENTED_EDGE('',*,*,#3917,.F.);
#5370=ORIENTED_EDGE('',*,*,#3918,.T.);
#5371=ORIENTED_EDGE('',*,*,#3919,.T.);
#5372=ORIENTED_EDGE('',*,*,#3920,.F.);
#5373=ORIENTED_EDGE('',*,*,#3921,.F.);
#5374=ORIENTED_EDGE('',*,*,#3922,.T.);
#5375=ORIENTED_EDGE('',*,*,#3923,.T.);
#5376=ORIENTED_EDGE('',*,*,#3918,.F.);
#5377=ORIENTED_EDGE('',*,*,#3924,.F.);
#5378=ORIENTED_EDGE('',*,*,#3925,.T.);
#5379=ORIENTED_EDGE('',*,*,#3926,.T.);
#5380=ORIENTED_EDGE('',*,*,#3922,.F.);
#5381=ORIENTED_EDGE('',*,*,#3927,.F.);
#5382=ORIENTED_EDGE('',*,*,#3928,.T.);
#5383=ORIENTED_EDGE('',*,*,#3929,.T.);
#5384=ORIENTED_EDGE('',*,*,#3925,.F.);
#5385=ORIENTED_EDGE('',*,*,#3930,.F.);
#5386=ORIENTED_EDGE('',*,*,#3931,.T.);
#5387=ORIENTED_EDGE('',*,*,#3932,.T.);
#5388=ORIENTED_EDGE('',*,*,#3928,.F.);
#5389=ORIENTED_EDGE('',*,*,#3933,.F.);
#5390=ORIENTED_EDGE('',*,*,#3920,.T.);
#5391=ORIENTED_EDGE('',*,*,#3934,.T.);
#5392=ORIENTED_EDGE('',*,*,#3931,.F.);
#5393=ORIENTED_EDGE('',*,*,#3934,.F.);
#5394=ORIENTED_EDGE('',*,*,#3919,.F.);
#5395=ORIENTED_EDGE('',*,*,#3923,.F.);
#5396=ORIENTED_EDGE('',*,*,#3926,.F.);
#5397=ORIENTED_EDGE('',*,*,#3929,.F.);
#5398=ORIENTED_EDGE('',*,*,#3932,.F.);
#5399=ORIENTED_EDGE('',*,*,#3935,.F.);
#5400=ORIENTED_EDGE('',*,*,#3936,.F.);
#5401=ORIENTED_EDGE('',*,*,#3937,.T.);
#5402=ORIENTED_EDGE('',*,*,#3938,.T.);
#5403=ORIENTED_EDGE('',*,*,#3939,.F.);
#5404=ORIENTED_EDGE('',*,*,#3940,.F.);
#5405=ORIENTED_EDGE('',*,*,#3941,.T.);
#5406=ORIENTED_EDGE('',*,*,#3942,.T.);
#5407=ORIENTED_EDGE('',*,*,#3937,.F.);
#5408=ORIENTED_EDGE('',*,*,#3943,.F.);
#5409=ORIENTED_EDGE('',*,*,#3944,.T.);
#5410=ORIENTED_EDGE('',*,*,#3945,.T.);
#5411=ORIENTED_EDGE('',*,*,#3941,.F.);
#5412=ORIENTED_EDGE('',*,*,#3946,.F.);
#5413=ORIENTED_EDGE('',*,*,#3947,.T.);
#5414=ORIENTED_EDGE('',*,*,#3948,.T.);
#5415=ORIENTED_EDGE('',*,*,#3944,.F.);
#5416=ORIENTED_EDGE('',*,*,#3949,.F.);
#5417=ORIENTED_EDGE('',*,*,#3950,.T.);
#5418=ORIENTED_EDGE('',*,*,#3951,.T.);
#5419=ORIENTED_EDGE('',*,*,#3947,.F.);
#5420=ORIENTED_EDGE('',*,*,#3952,.F.);
#5421=ORIENTED_EDGE('',*,*,#3939,.T.);
#5422=ORIENTED_EDGE('',*,*,#3953,.T.);
#5423=ORIENTED_EDGE('',*,*,#3950,.F.);
#5424=ORIENTED_EDGE('',*,*,#3953,.F.);
#5425=ORIENTED_EDGE('',*,*,#3938,.F.);
#5426=ORIENTED_EDGE('',*,*,#3942,.F.);
#5427=ORIENTED_EDGE('',*,*,#3945,.F.);
#5428=ORIENTED_EDGE('',*,*,#3948,.F.);
#5429=ORIENTED_EDGE('',*,*,#3951,.F.);
#5430=ORIENTED_EDGE('',*,*,#3954,.F.);
#5431=ORIENTED_EDGE('',*,*,#3954,.T.);
#5432=ORIENTED_EDGE('',*,*,#3955,.T.);
#5433=ORIENTED_EDGE('',*,*,#3956,.F.);
#5434=ORIENTED_EDGE('',*,*,#3955,.F.);
#5435=ORIENTED_EDGE('',*,*,#3935,.T.);
#5436=ORIENTED_EDGE('',*,*,#3957,.T.);
#5437=ORIENTED_EDGE('',*,*,#3958,.F.);
#5438=ORIENTED_EDGE('',*,*,#3957,.F.);
#5439=ORIENTED_EDGE('',*,*,#3959,.F.);
#5440=ORIENTED_EDGE('',*,*,#3960,.F.);
#5441=ORIENTED_EDGE('',*,*,#3961,.F.);
#5442=ORIENTED_EDGE('',*,*,#3962,.T.);
#5443=ORIENTED_EDGE('',*,*,#3963,.F.);
#5444=ORIENTED_EDGE('',*,*,#3964,.T.);
#5445=ORIENTED_EDGE('',*,*,#3965,.F.);
#5446=ORIENTED_EDGE('',*,*,#3966,.F.);
#5447=ORIENTED_EDGE('',*,*,#3967,.F.);
#5448=ORIENTED_EDGE('',*,*,#3968,.T.);
#5449=ORIENTED_EDGE('',*,*,#3969,.F.);
#5450=ORIENTED_EDGE('',*,*,#3970,.F.);
#5451=ORIENTED_EDGE('',*,*,#3971,.F.);
#5452=ORIENTED_EDGE('',*,*,#3972,.T.);
#5453=ORIENTED_EDGE('',*,*,#3973,.F.);
#5454=ORIENTED_EDGE('',*,*,#3974,.F.);
#5455=ORIENTED_EDGE('',*,*,#3975,.F.);
#5456=ORIENTED_EDGE('',*,*,#3976,.T.);
#5457=ORIENTED_EDGE('',*,*,#3977,.F.);
#5458=ORIENTED_EDGE('',*,*,#3978,.F.);
#5459=ORIENTED_EDGE('',*,*,#3979,.F.);
#5460=ORIENTED_EDGE('',*,*,#3980,.F.);
#5461=ORIENTED_EDGE('',*,*,#3981,.F.);
#5462=ORIENTED_EDGE('',*,*,#3982,.T.);
#5463=ORIENTED_EDGE('',*,*,#3983,.F.);
#5464=ORIENTED_EDGE('',*,*,#3984,.F.);
#5465=ORIENTED_EDGE('',*,*,#3985,.F.);
#5466=ORIENTED_EDGE('',*,*,#3986,.T.);
#5467=ORIENTED_EDGE('',*,*,#3987,.F.);
#5468=ORIENTED_EDGE('',*,*,#3956,.T.);
#5469=ORIENTED_EDGE('',*,*,#3988,.F.);
#5470=ORIENTED_EDGE('',*,*,#3958,.T.);
#5471=ORIENTED_EDGE('',*,*,#3989,.F.);
#5472=ORIENTED_EDGE('',*,*,#3962,.F.);
#5473=ORIENTED_EDGE('',*,*,#3990,.F.);
#5474=ORIENTED_EDGE('',*,*,#3976,.F.);
#5475=ORIENTED_EDGE('',*,*,#3991,.F.);
#5476=ORIENTED_EDGE('',*,*,#3982,.F.);
#5477=ORIENTED_EDGE('',*,*,#3992,.F.);
#5478=ORIENTED_EDGE('',*,*,#3964,.F.);
#5479=ORIENTED_EDGE('',*,*,#3993,.F.);
#5480=ORIENTED_EDGE('',*,*,#3986,.F.);
#5481=ORIENTED_EDGE('',*,*,#3994,.F.);
#5482=ORIENTED_EDGE('',*,*,#3968,.F.);
#5483=ORIENTED_EDGE('',*,*,#3995,.F.);
#5484=ORIENTED_EDGE('',*,*,#3996,.F.);
#5485=ORIENTED_EDGE('',*,*,#3997,.F.);
#5486=ORIENTED_EDGE('',*,*,#3972,.F.);
#5487=ORIENTED_EDGE('',*,*,#3998,.F.);
#5488=ORIENTED_EDGE('',*,*,#3999,.F.);
#5489=ORIENTED_EDGE('',*,*,#4000,.F.);
#5490=ORIENTED_EDGE('',*,*,#3996,.T.);
#5491=ORIENTED_EDGE('',*,*,#4001,.T.);
#5492=ORIENTED_EDGE('',*,*,#4002,.F.);
#5493=ORIENTED_EDGE('',*,*,#4003,.F.);
#5494=ORIENTED_EDGE('',*,*,#4004,.F.);
#5495=ORIENTED_EDGE('',*,*,#4005,.F.);
#5496=ORIENTED_EDGE('',*,*,#4006,.F.);
#5497=ORIENTED_EDGE('',*,*,#3973,.T.);
#5498=ORIENTED_EDGE('',*,*,#3997,.T.);
#5499=ORIENTED_EDGE('',*,*,#4000,.T.);
#5500=ORIENTED_EDGE('',*,*,#4007,.T.);
#5501=ORIENTED_EDGE('',*,*,#4008,.F.);
#5502=ORIENTED_EDGE('',*,*,#4009,.F.);
#5503=ORIENTED_EDGE('',*,*,#4010,.F.);
#5504=ORIENTED_EDGE('',*,*,#4011,.F.);
#5505=ORIENTED_EDGE('',*,*,#4012,.F.);
#5506=ORIENTED_EDGE('',*,*,#4013,.T.);
#5507=ORIENTED_EDGE('',*,*,#3969,.T.);
#5508=ORIENTED_EDGE('',*,*,#3994,.T.);
#5509=ORIENTED_EDGE('',*,*,#3985,.T.);
#5510=ORIENTED_EDGE('',*,*,#4014,.T.);
#5511=ORIENTED_EDGE('',*,*,#4015,.F.);
#5512=ORIENTED_EDGE('',*,*,#4016,.F.);
#5513=ORIENTED_EDGE('',*,*,#4017,.F.);
#5514=ORIENTED_EDGE('',*,*,#4018,.F.);
#5515=ORIENTED_EDGE('',*,*,#4019,.F.);
#5516=ORIENTED_EDGE('',*,*,#4020,.T.);
#5517=ORIENTED_EDGE('',*,*,#3965,.T.);
#5518=ORIENTED_EDGE('',*,*,#3992,.T.);
#5519=ORIENTED_EDGE('',*,*,#3981,.T.);
#5520=ORIENTED_EDGE('',*,*,#4021,.T.);
#5521=ORIENTED_EDGE('',*,*,#4022,.F.);
#5522=ORIENTED_EDGE('',*,*,#4023,.F.);
#5523=ORIENTED_EDGE('',*,*,#3901,.F.);
#5524=ORIENTED_EDGE('',*,*,#4024,.F.);
#5525=ORIENTED_EDGE('',*,*,#4025,.F.);
#5526=ORIENTED_EDGE('',*,*,#4026,.T.);
#5527=ORIENTED_EDGE('',*,*,#3959,.T.);
#5528=ORIENTED_EDGE('',*,*,#3989,.T.);
#5529=ORIENTED_EDGE('',*,*,#3975,.T.);
#5530=ORIENTED_EDGE('',*,*,#4027,.F.);
#5531=ORIENTED_EDGE('',*,*,#4028,.T.);
#5532=ORIENTED_EDGE('',*,*,#4029,.T.);
#5533=ORIENTED_EDGE('',*,*,#4030,.T.);
#5534=ORIENTED_EDGE('',*,*,#4031,.F.);
#5535=ORIENTED_EDGE('',*,*,#3974,.T.);
#5536=ORIENTED_EDGE('',*,*,#4013,.F.);
#5537=ORIENTED_EDGE('',*,*,#4032,.T.);
#5538=ORIENTED_EDGE('',*,*,#4001,.F.);
#5539=ORIENTED_EDGE('',*,*,#4033,.T.);
#5540=ORIENTED_EDGE('',*,*,#4007,.F.);
#5541=ORIENTED_EDGE('',*,*,#3999,.T.);
#5542=ORIENTED_EDGE('',*,*,#4034,.F.);
#5543=ORIENTED_EDGE('',*,*,#4035,.T.);
#5544=ORIENTED_EDGE('',*,*,#4014,.F.);
#5545=ORIENTED_EDGE('',*,*,#3984,.T.);
#5546=ORIENTED_EDGE('',*,*,#4036,.F.);
#5547=ORIENTED_EDGE('',*,*,#4037,.T.);
#5548=ORIENTED_EDGE('',*,*,#4021,.F.);
#5549=ORIENTED_EDGE('',*,*,#3980,.T.);
#5550=ORIENTED_EDGE('',*,*,#4038,.F.);
#5551=ORIENTED_EDGE('',*,*,#4039,.T.);
#5552=ORIENTED_EDGE('',*,*,#4040,.T.);
#5553=ORIENTED_EDGE('',*,*,#4027,.T.);
#5554=ORIENTED_EDGE('',*,*,#3978,.T.);
#5555=ORIENTED_EDGE('',*,*,#4041,.T.);
#5556=ORIENTED_EDGE('',*,*,#4042,.F.);
#5557=ORIENTED_EDGE('',*,*,#4043,.T.);
#5558=ORIENTED_EDGE('',*,*,#4044,.F.);
#5559=ORIENTED_EDGE('',*,*,#4045,.T.);
#5560=ORIENTED_EDGE('',*,*,#4046,.F.);
#5561=ORIENTED_EDGE('',*,*,#4047,.T.);
#5562=ORIENTED_EDGE('',*,*,#4048,.F.);
#5563=ORIENTED_EDGE('',*,*,#4049,.T.);
#5564=ORIENTED_EDGE('',*,*,#3960,.T.);
#5565=ORIENTED_EDGE('',*,*,#4031,.T.);
#5566=ORIENTED_EDGE('',*,*,#4050,.T.);
#5567=ORIENTED_EDGE('',*,*,#4051,.T.);
#5568=ORIENTED_EDGE('',*,*,#4052,.F.);
#5569=ORIENTED_EDGE('',*,*,#3966,.T.);
#5570=ORIENTED_EDGE('',*,*,#4026,.F.);
#5571=ORIENTED_EDGE('',*,*,#4053,.T.);
#5572=ORIENTED_EDGE('',*,*,#4054,.F.);
#5573=ORIENTED_EDGE('',*,*,#3970,.T.);
#5574=ORIENTED_EDGE('',*,*,#4020,.F.);
#5575=ORIENTED_EDGE('',*,*,#4055,.T.);
#5576=ORIENTED_EDGE('',*,*,#4056,.F.);
#5577=ORIENTED_EDGE('',*,*,#4057,.T.);
#5578=ORIENTED_EDGE('',*,*,#4058,.T.);
#5579=ORIENTED_EDGE('',*,*,#4059,.T.);
#5580=ORIENTED_EDGE('',*,*,#4060,.T.);
#5581=ORIENTED_EDGE('',*,*,#4061,.T.);
#5582=ORIENTED_EDGE('',*,*,#4062,.F.);
#5583=ORIENTED_EDGE('',*,*,#4063,.F.);
#5584=ORIENTED_EDGE('',*,*,#4064,.T.);
#5585=ORIENTED_EDGE('',*,*,#3988,.T.);
#5586=ORIENTED_EDGE('',*,*,#4064,.F.);
#5587=ORIENTED_EDGE('',*,*,#3906,.F.);
#5588=ORIENTED_EDGE('',*,*,#4065,.T.);
#5589=ORIENTED_EDGE('',*,*,#3987,.T.);
#5590=ORIENTED_EDGE('',*,*,#4065,.F.);
#5591=ORIENTED_EDGE('',*,*,#4066,.F.);
#5592=ORIENTED_EDGE('',*,*,#4062,.T.);
#5593=ORIENTED_EDGE('',*,*,#4067,.F.);
#5594=ORIENTED_EDGE('',*,*,#4068,.F.);
#5595=ORIENTED_EDGE('',*,*,#4069,.F.);
#5596=ORIENTED_EDGE('',*,*,#4070,.F.);
#5597=ORIENTED_EDGE('',*,*,#4002,.T.);
#5598=ORIENTED_EDGE('',*,*,#4032,.F.);
#5599=ORIENTED_EDGE('',*,*,#4012,.T.);
#5600=ORIENTED_EDGE('',*,*,#4071,.T.);
#5601=ORIENTED_EDGE('',*,*,#4066,.T.);
#5602=ORIENTED_EDGE('',*,*,#4072,.T.);
#5603=ORIENTED_EDGE('',*,*,#4073,.T.);
#5604=ORIENTED_EDGE('',*,*,#4057,.F.);
#5605=ORIENTED_EDGE('',*,*,#4003,.T.);
#5606=ORIENTED_EDGE('',*,*,#4071,.F.);
#5607=ORIENTED_EDGE('',*,*,#4011,.T.);
#5608=ORIENTED_EDGE('',*,*,#4074,.F.);
#5609=ORIENTED_EDGE('',*,*,#4070,.T.);
#5610=ORIENTED_EDGE('',*,*,#4075,.F.);
#5611=ORIENTED_EDGE('',*,*,#4076,.F.);
#5612=ORIENTED_EDGE('',*,*,#4072,.F.);
#5613=ORIENTED_EDGE('',*,*,#4004,.T.);
#5614=ORIENTED_EDGE('',*,*,#4074,.T.);
#5615=ORIENTED_EDGE('',*,*,#4010,.T.);
#5616=ORIENTED_EDGE('',*,*,#4077,.T.);
#5617=ORIENTED_EDGE('',*,*,#3909,.T.);
#5618=ORIENTED_EDGE('',*,*,#3916,.T.);
#5619=ORIENTED_EDGE('',*,*,#4063,.T.);
#5620=ORIENTED_EDGE('',*,*,#4069,.T.);
#5621=ORIENTED_EDGE('',*,*,#4078,.T.);
#5622=ORIENTED_EDGE('',*,*,#4079,.T.);
#5623=ORIENTED_EDGE('',*,*,#4075,.T.);
#5624=ORIENTED_EDGE('',*,*,#4005,.T.);
#5625=ORIENTED_EDGE('',*,*,#4077,.F.);
#5626=ORIENTED_EDGE('',*,*,#4009,.T.);
#5627=ORIENTED_EDGE('',*,*,#4080,.F.);
#5628=ORIENTED_EDGE('',*,*,#4006,.T.);
#5629=ORIENTED_EDGE('',*,*,#4080,.T.);
#5630=ORIENTED_EDGE('',*,*,#4008,.T.);
#5631=ORIENTED_EDGE('',*,*,#4033,.F.);
#5632=ORIENTED_EDGE('',*,*,#4067,.T.);
#5633=ORIENTED_EDGE('',*,*,#4061,.F.);
#5634=ORIENTED_EDGE('',*,*,#4081,.T.);
#5635=ORIENTED_EDGE('',*,*,#4082,.T.);
#5636=ORIENTED_EDGE('',*,*,#3971,.T.);
#5637=ORIENTED_EDGE('',*,*,#4056,.T.);
#5638=ORIENTED_EDGE('',*,*,#4083,.F.);
#5639=ORIENTED_EDGE('',*,*,#4084,.F.);
#5640=ORIENTED_EDGE('',*,*,#4085,.F.);
#5641=ORIENTED_EDGE('',*,*,#4086,.F.);
#5642=ORIENTED_EDGE('',*,*,#4087,.F.);
#5643=ORIENTED_EDGE('',*,*,#4034,.T.);
#5644=ORIENTED_EDGE('',*,*,#3998,.T.);
#5645=ORIENTED_EDGE('',*,*,#3995,.T.);
#5646=ORIENTED_EDGE('',*,*,#4083,.T.);
#5647=ORIENTED_EDGE('',*,*,#4055,.F.);
#5648=ORIENTED_EDGE('',*,*,#4019,.T.);
#5649=ORIENTED_EDGE('',*,*,#4088,.T.);
#5650=ORIENTED_EDGE('',*,*,#4084,.T.);
#5651=ORIENTED_EDGE('',*,*,#4088,.F.);
#5652=ORIENTED_EDGE('',*,*,#4018,.T.);
#5653=ORIENTED_EDGE('',*,*,#4089,.F.);
#5654=ORIENTED_EDGE('',*,*,#4085,.T.);
#5655=ORIENTED_EDGE('',*,*,#4089,.T.);
#5656=ORIENTED_EDGE('',*,*,#4017,.T.);
#5657=ORIENTED_EDGE('',*,*,#4090,.T.);
#5658=ORIENTED_EDGE('',*,*,#4086,.T.);
#5659=ORIENTED_EDGE('',*,*,#4090,.F.);
#5660=ORIENTED_EDGE('',*,*,#4016,.T.);
#5661=ORIENTED_EDGE('',*,*,#4091,.F.);
#5662=ORIENTED_EDGE('',*,*,#4087,.T.);
#5663=ORIENTED_EDGE('',*,*,#4091,.T.);
#5664=ORIENTED_EDGE('',*,*,#4015,.T.);
#5665=ORIENTED_EDGE('',*,*,#4035,.F.);
#5666=ORIENTED_EDGE('',*,*,#3967,.T.);
#5667=ORIENTED_EDGE('',*,*,#4054,.T.);
#5668=ORIENTED_EDGE('',*,*,#4092,.F.);
#5669=ORIENTED_EDGE('',*,*,#4093,.F.);
#5670=ORIENTED_EDGE('',*,*,#3897,.F.);
#5671=ORIENTED_EDGE('',*,*,#4094,.F.);
#5672=ORIENTED_EDGE('',*,*,#4095,.F.);
#5673=ORIENTED_EDGE('',*,*,#4036,.T.);
#5674=ORIENTED_EDGE('',*,*,#3983,.T.);
#5675=ORIENTED_EDGE('',*,*,#3993,.T.);
#5676=ORIENTED_EDGE('',*,*,#4092,.T.);
#5677=ORIENTED_EDGE('',*,*,#4053,.F.);
#5678=ORIENTED_EDGE('',*,*,#4025,.T.);
#5679=ORIENTED_EDGE('',*,*,#4096,.T.);
#5680=ORIENTED_EDGE('',*,*,#3899,.T.);
#5681=ORIENTED_EDGE('',*,*,#3898,.F.);
#5682=ORIENTED_EDGE('',*,*,#4093,.T.);
#5683=ORIENTED_EDGE('',*,*,#4096,.F.);
#5684=ORIENTED_EDGE('',*,*,#4024,.T.);
#5685=ORIENTED_EDGE('',*,*,#3900,.F.);
#5686=ORIENTED_EDGE('',*,*,#3903,.T.);
#5687=ORIENTED_EDGE('',*,*,#3902,.F.);
#5688=ORIENTED_EDGE('',*,*,#4023,.T.);
#5689=ORIENTED_EDGE('',*,*,#4097,.F.);
#5690=ORIENTED_EDGE('',*,*,#4094,.T.);
#5691=ORIENTED_EDGE('',*,*,#3896,.F.);
#5692=ORIENTED_EDGE('',*,*,#4095,.T.);
#5693=ORIENTED_EDGE('',*,*,#4097,.T.);
#5694=ORIENTED_EDGE('',*,*,#4022,.T.);
#5695=ORIENTED_EDGE('',*,*,#4037,.F.);
#5696=ORIENTED_EDGE('',*,*,#3963,.T.);
#5697=ORIENTED_EDGE('',*,*,#4052,.T.);
#5698=ORIENTED_EDGE('',*,*,#4098,.F.);
#5699=ORIENTED_EDGE('',*,*,#4099,.F.);
#5700=ORIENTED_EDGE('',*,*,#4100,.F.);
#5701=ORIENTED_EDGE('',*,*,#4101,.F.);
#5702=ORIENTED_EDGE('',*,*,#4102,.F.);
#5703=ORIENTED_EDGE('',*,*,#4038,.T.);
#5704=ORIENTED_EDGE('',*,*,#3979,.T.);
#5705=ORIENTED_EDGE('',*,*,#3991,.T.);
#5706=ORIENTED_EDGE('',*,*,#4098,.T.);
#5707=ORIENTED_EDGE('',*,*,#4051,.F.);
#5708=ORIENTED_EDGE('',*,*,#4103,.T.);
#5709=ORIENTED_EDGE('',*,*,#4104,.T.);
#5710=ORIENTED_EDGE('',*,*,#4099,.T.);
#5711=ORIENTED_EDGE('',*,*,#4104,.F.);
#5712=ORIENTED_EDGE('',*,*,#4105,.F.);
#5713=ORIENTED_EDGE('',*,*,#4106,.F.);
#5714=ORIENTED_EDGE('',*,*,#4100,.T.);
#5715=ORIENTED_EDGE('',*,*,#4106,.T.);
#5716=ORIENTED_EDGE('',*,*,#4107,.T.);
#5717=ORIENTED_EDGE('',*,*,#4108,.T.);
#5718=ORIENTED_EDGE('',*,*,#4102,.T.);
#5719=ORIENTED_EDGE('',*,*,#4109,.T.);
#5720=ORIENTED_EDGE('',*,*,#4110,.T.);
#5721=ORIENTED_EDGE('',*,*,#4039,.F.);
#5722=ORIENTED_EDGE('',*,*,#4101,.T.);
#5723=ORIENTED_EDGE('',*,*,#4108,.F.);
#5724=ORIENTED_EDGE('',*,*,#4111,.F.);
#5725=ORIENTED_EDGE('',*,*,#4109,.F.);
#5726=ORIENTED_EDGE('',*,*,#4112,.T.);
#5727=ORIENTED_EDGE('',*,*,#4113,.T.);
#5728=ORIENTED_EDGE('',*,*,#4111,.T.);
#5729=ORIENTED_EDGE('',*,*,#4114,.T.);
#5730=ORIENTED_EDGE('',*,*,#4115,.T.);
#5731=ORIENTED_EDGE('',*,*,#4116,.T.);
#5732=ORIENTED_EDGE('',*,*,#4105,.T.);
#5733=ORIENTED_EDGE('',*,*,#4117,.T.);
#5734=ORIENTED_EDGE('',*,*,#4118,.T.);
#5735=ORIENTED_EDGE('',*,*,#4112,.F.);
#5736=ORIENTED_EDGE('',*,*,#4107,.F.);
#5737=ORIENTED_EDGE('',*,*,#4118,.F.);
#5738=ORIENTED_EDGE('',*,*,#4029,.F.);
#5739=ORIENTED_EDGE('',*,*,#4050,.F.);
#5740=ORIENTED_EDGE('',*,*,#4030,.F.);
#5741=ORIENTED_EDGE('',*,*,#4117,.F.);
#5742=ORIENTED_EDGE('',*,*,#4103,.F.);
#5743=ORIENTED_EDGE('',*,*,#4119,.T.);
#5744=ORIENTED_EDGE('',*,*,#4076,.T.);
#5745=ORIENTED_EDGE('',*,*,#4120,.T.);
#5746=ORIENTED_EDGE('',*,*,#4120,.F.);
#5747=ORIENTED_EDGE('',*,*,#4079,.F.);
#5748=ORIENTED_EDGE('',*,*,#4116,.F.);
#5749=ORIENTED_EDGE('',*,*,#4121,.F.);
#5750=ORIENTED_EDGE('',*,*,#4058,.F.);
#5751=ORIENTED_EDGE('',*,*,#4073,.F.);
#5752=ORIENTED_EDGE('',*,*,#4119,.F.);
#5753=ORIENTED_EDGE('',*,*,#4122,.F.);
#5754=ORIENTED_EDGE('',*,*,#4060,.F.);
#5755=ORIENTED_EDGE('',*,*,#4123,.F.);
#5756=ORIENTED_EDGE('',*,*,#4115,.F.);
#5757=ORIENTED_EDGE('',*,*,#4081,.F.);
#5758=ORIENTED_EDGE('',*,*,#4068,.T.);
#5759=ORIENTED_EDGE('',*,*,#4082,.F.);
#5760=ORIENTED_EDGE('',*,*,#4114,.F.);
#5761=ORIENTED_EDGE('',*,*,#4078,.F.);
#5762=ORIENTED_EDGE('',*,*,#4040,.F.);
#5763=ORIENTED_EDGE('',*,*,#4110,.F.);
#5764=ORIENTED_EDGE('',*,*,#4113,.F.);
#5765=ORIENTED_EDGE('',*,*,#4028,.F.);
#5766=ORIENTED_EDGE('',*,*,#4122,.T.);
#5767=ORIENTED_EDGE('',*,*,#4121,.T.);
#5768=ORIENTED_EDGE('',*,*,#4123,.T.);
#5769=ORIENTED_EDGE('',*,*,#4059,.F.);
#5770=ORIENTED_EDGE('',*,*,#4124,.F.);
#5771=ORIENTED_EDGE('',*,*,#4125,.F.);
#5772=ORIENTED_EDGE('',*,*,#4126,.F.);
#5773=ORIENTED_EDGE('',*,*,#4127,.F.);
#5774=ORIENTED_EDGE('',*,*,#4128,.F.);
#5775=ORIENTED_EDGE('',*,*,#4129,.F.);
#5776=ORIENTED_EDGE('',*,*,#4130,.F.);
#5777=ORIENTED_EDGE('',*,*,#4131,.F.);
#5778=ORIENTED_EDGE('',*,*,#4132,.F.);
#5779=ORIENTED_EDGE('',*,*,#4124,.T.);
#5780=ORIENTED_EDGE('',*,*,#4133,.T.);
#5781=ORIENTED_EDGE('',*,*,#4131,.T.);
#5782=ORIENTED_EDGE('',*,*,#4134,.T.);
#5783=ORIENTED_EDGE('',*,*,#4048,.T.);
#5784=ORIENTED_EDGE('',*,*,#4135,.T.);
#5785=ORIENTED_EDGE('',*,*,#4132,.T.);
#5786=ORIENTED_EDGE('',*,*,#4136,.T.);
#5787=ORIENTED_EDGE('',*,*,#4137,.F.);
#5788=ORIENTED_EDGE('',*,*,#4138,.F.);
#5789=ORIENTED_EDGE('',*,*,#4139,.F.);
#5790=ORIENTED_EDGE('',*,*,#4138,.T.);
#5791=ORIENTED_EDGE('',*,*,#4140,.T.);
#5792=ORIENTED_EDGE('',*,*,#4128,.T.);
#5793=ORIENTED_EDGE('',*,*,#4141,.T.);
#5794=ORIENTED_EDGE('',*,*,#4130,.T.);
#5795=ORIENTED_EDGE('',*,*,#4142,.T.);
#5796=ORIENTED_EDGE('',*,*,#4139,.T.);
#5797=ORIENTED_EDGE('',*,*,#4143,.T.);
#5798=ORIENTED_EDGE('',*,*,#4046,.T.);
#5799=ORIENTED_EDGE('',*,*,#4144,.T.);
#5800=ORIENTED_EDGE('',*,*,#4137,.T.);
#5801=ORIENTED_EDGE('',*,*,#4145,.T.);
#5802=ORIENTED_EDGE('',*,*,#4044,.T.);
#5803=ORIENTED_EDGE('',*,*,#4146,.T.);
#5804=ORIENTED_EDGE('',*,*,#4129,.T.);
#5805=ORIENTED_EDGE('',*,*,#4147,.T.);
#5806=ORIENTED_EDGE('',*,*,#4127,.T.);
#5807=ORIENTED_EDGE('',*,*,#4148,.T.);
#5808=ORIENTED_EDGE('',*,*,#4125,.T.);
#5809=ORIENTED_EDGE('',*,*,#4149,.T.);
#5810=ORIENTED_EDGE('',*,*,#4042,.T.);
#5811=ORIENTED_EDGE('',*,*,#4150,.T.);
#5812=ORIENTED_EDGE('',*,*,#4126,.T.);
#5813=ORIENTED_EDGE('',*,*,#4151,.T.);
#5814=ORIENTED_EDGE('',*,*,#4145,.F.);
#5815=ORIENTED_EDGE('',*,*,#4142,.F.);
#5816=ORIENTED_EDGE('',*,*,#4135,.F.);
#5817=ORIENTED_EDGE('',*,*,#4047,.F.);
#5818=ORIENTED_EDGE('',*,*,#3961,.T.);
#5819=ORIENTED_EDGE('',*,*,#4049,.F.);
#5820=ORIENTED_EDGE('',*,*,#4136,.F.);
#5821=ORIENTED_EDGE('',*,*,#4133,.F.);
#5822=ORIENTED_EDGE('',*,*,#4150,.F.);
#5823=ORIENTED_EDGE('',*,*,#4041,.F.);
#5824=ORIENTED_EDGE('',*,*,#3977,.T.);
#5825=ORIENTED_EDGE('',*,*,#3990,.T.);
#5826=ORIENTED_EDGE('',*,*,#4141,.F.);
#5827=ORIENTED_EDGE('',*,*,#4149,.F.);
#5828=ORIENTED_EDGE('',*,*,#4134,.F.);
#5829=ORIENTED_EDGE('',*,*,#4143,.F.);
#5830=ORIENTED_EDGE('',*,*,#3936,.T.);
#5831=ORIENTED_EDGE('',*,*,#3952,.T.);
#5832=ORIENTED_EDGE('',*,*,#3949,.T.);
#5833=ORIENTED_EDGE('',*,*,#3946,.T.);
#5834=ORIENTED_EDGE('',*,*,#3943,.T.);
#5835=ORIENTED_EDGE('',*,*,#3940,.T.);
#5836=ORIENTED_EDGE('',*,*,#3917,.T.);
#5837=ORIENTED_EDGE('',*,*,#3933,.T.);
#5838=ORIENTED_EDGE('',*,*,#3930,.T.);
#5839=ORIENTED_EDGE('',*,*,#3927,.T.);
#5840=ORIENTED_EDGE('',*,*,#3924,.T.);
#5841=ORIENTED_EDGE('',*,*,#3921,.T.);
#5842=ORIENTED_EDGE('',*,*,#3914,.T.);
#5843=ORIENTED_EDGE('',*,*,#3912,.T.);
#5844=ORIENTED_EDGE('',*,*,#3910,.T.);
#5845=ORIENTED_EDGE('',*,*,#3907,.T.);
#5846=ORIENTED_EDGE('',*,*,#4146,.F.);
#5847=ORIENTED_EDGE('',*,*,#4043,.F.);
#5848=ORIENTED_EDGE('',*,*,#4151,.F.);
#5849=ORIENTED_EDGE('',*,*,#4148,.F.);
#5850=ORIENTED_EDGE('',*,*,#4144,.F.);
#5851=ORIENTED_EDGE('',*,*,#4045,.F.);
#5852=ORIENTED_EDGE('',*,*,#4147,.F.);
#5853=ORIENTED_EDGE('',*,*,#4140,.F.);
#6599=CYLINDRICAL_SURFACE('',#7480,0.15);
#6600=CYLINDRICAL_SURFACE('',#7483,0.15);
#6601=CYLINDRICAL_SURFACE('',#7485,0.15);
#6602=CYLINDRICAL_SURFACE('',#7487,0.15);
#6603=CYLINDRICAL_SURFACE('',#7506,0.17);
#6604=CYLINDRICAL_SURFACE('',#7508,0.17);
#6605=CYLINDRICAL_SURFACE('',#7532,0.4);
#6606=CYLINDRICAL_SURFACE('',#7534,0.4);
#6607=CYLINDRICAL_SURFACE('',#7556,0.1);
#6608=CYLINDRICAL_SURFACE('',#7560,0.1);
#6609=CYLINDRICAL_SURFACE('',#7574,0.3);
#6610=CYLINDRICAL_SURFACE('',#7579,0.3);
#6866=ADVANCED_FACE('',(#987,#625,#626,#627),#742,.F.);
#6867=ADVANCED_FACE('',(#988),#6599,.F.);
#6868=ADVANCED_FACE('',(#989),#6600,.F.);
#6869=ADVANCED_FACE('',(#990),#6601,.F.);
#6870=ADVANCED_FACE('',(#991),#6602,.F.);
#6871=ADVANCED_FACE('',(#992),#743,.F.);
#6872=ADVANCED_FACE('',(#993),#744,.F.);
#6873=ADVANCED_FACE('',(#994),#745,.F.);
#6874=ADVANCED_FACE('',(#995),#746,.F.);
#6875=ADVANCED_FACE('',(#996),#747,.F.);
#6876=ADVANCED_FACE('',(#997),#748,.F.);
#6877=ADVANCED_FACE('',(#998,#628),#749,.F.);
#6878=ADVANCED_FACE('',(#999),#750,.F.);
#6879=ADVANCED_FACE('',(#1000),#751,.F.);
#6880=ADVANCED_FACE('',(#1001),#752,.F.);
#6881=ADVANCED_FACE('',(#1002),#753,.F.);
#6882=ADVANCED_FACE('',(#1003),#754,.F.);
#6883=ADVANCED_FACE('',(#1004),#755,.F.);
#6884=ADVANCED_FACE('',(#1005,#629),#756,.F.);
#6885=ADVANCED_FACE('',(#1006),#6603,.F.);
#6886=ADVANCED_FACE('',(#1007),#6604,.F.);
#6887=ADVANCED_FACE('',(#1008),#757,.F.);
#6888=ADVANCED_FACE('',(#1009),#758,.F.);
#6889=ADVANCED_FACE('',(#1010),#759,.F.);
#6890=ADVANCED_FACE('',(#1011),#760,.F.);
#6891=ADVANCED_FACE('',(#1012),#761,.F.);
#6892=ADVANCED_FACE('',(#1013),#762,.F.);
#6893=ADVANCED_FACE('',(#1014),#763,.F.);
#6894=ADVANCED_FACE('',(#1015,#630),#764,.F.);
#6895=ADVANCED_FACE('',(#1016,#631),#765,.F.);
#6896=ADVANCED_FACE('',(#1017),#766,.F.);
#6897=ADVANCED_FACE('',(#1018),#767,.F.);
#6898=ADVANCED_FACE('',(#1019),#768,.F.);
#6899=ADVANCED_FACE('',(#1020),#769,.F.);
#6900=ADVANCED_FACE('',(#1021),#770,.F.);
#6901=ADVANCED_FACE('',(#1022),#771,.T.);
#6902=ADVANCED_FACE('',(#1023),#772,.T.);
#6903=ADVANCED_FACE('',(#1024),#773,.T.);
#6904=ADVANCED_FACE('',(#1025),#774,.T.);
#6905=ADVANCED_FACE('',(#1026),#775,.T.);
#6906=ADVANCED_FACE('',(#1027,#632),#776,.F.);
#6907=ADVANCED_FACE('',(#1028),#6605,.T.);
#6908=ADVANCED_FACE('',(#1029),#6606,.T.);
#6909=ADVANCED_FACE('',(#1030),#777,.T.);
#6910=ADVANCED_FACE('',(#1031),#123,.T.);
#6911=ADVANCED_FACE('',(#1032),#124,.T.);
#6912=ADVANCED_FACE('',(#1033),#125,.T.);
#6913=ADVANCED_FACE('',(#1034),#126,.T.);
#6914=ADVANCED_FACE('',(#1035,#633,#634,#635),#778,.F.);
#6915=ADVANCED_FACE('',(#1036),#779,.F.);
#6916=ADVANCED_FACE('',(#1037),#127,.T.);
#6917=ADVANCED_FACE('',(#1038),#128,.T.);
#6918=ADVANCED_FACE('',(#1039),#129,.T.);
#6919=ADVANCED_FACE('',(#1040),#780,.T.);
#6920=ADVANCED_FACE('',(#1041),#130,.T.);
#6921=ADVANCED_FACE('',(#1042),#131,.T.);
#6922=ADVANCED_FACE('',(#1043),#781,.F.);
#6923=ADVANCED_FACE('',(#1044),#132,.T.);
#6924=ADVANCED_FACE('',(#1045),#133,.T.);
#6925=ADVANCED_FACE('',(#1046),#782,.T.);
#6926=ADVANCED_FACE('',(#1047),#134,.T.);
#6927=ADVANCED_FACE('',(#1048),#135,.T.);
#6928=ADVANCED_FACE('',(#1049),#136,.T.);
#6929=ADVANCED_FACE('',(#1050),#137,.T.);
#6930=ADVANCED_FACE('',(#1051),#783,.T.);
#6931=ADVANCED_FACE('',(#1052),#138,.T.);
#6932=ADVANCED_FACE('',(#1053),#139,.T.);
#6933=ADVANCED_FACE('',(#1054),#784,.F.);
#6934=ADVANCED_FACE('',(#1055),#140,.T.);
#6935=ADVANCED_FACE('',(#1056),#141,.T.);
#6936=ADVANCED_FACE('',(#1057),#83,.F.);
#6937=ADVANCED_FACE('',(#1058),#84,.F.);
#6938=ADVANCED_FACE('',(#1059),#85,.F.);
#6939=ADVANCED_FACE('',(#1060),#6607,.F.);
#6940=ADVANCED_FACE('',(#1061),#142,.T.);
#6941=ADVANCED_FACE('',(#1062),#86,.F.);
#6942=ADVANCED_FACE('',(#1063),#6608,.F.);
#6943=ADVANCED_FACE('',(#1064),#143,.T.);
#6944=ADVANCED_FACE('',(#1065),#144,.T.);
#6945=ADVANCED_FACE('',(#1066),#145,.T.);
#6946=ADVANCED_FACE('',(#1067),#146,.T.);
#6947=ADVANCED_FACE('',(#1068),#785,.T.);
#6948=ADVANCED_FACE('',(#1069),#87,.T.);
#6949=ADVANCED_FACE('',(#1070),#88,.T.);
#6950=ADVANCED_FACE('',(#1071),#89,.T.);
#6951=ADVANCED_FACE('',(#1072),#6609,.T.);
#6952=ADVANCED_FACE('',(#1073),#147,.F.);
#6953=ADVANCED_FACE('',(#1074),#90,.T.);
#6954=ADVANCED_FACE('',(#1075),#6610,.T.);
#6955=ADVANCED_FACE('',(#1076),#148,.F.);
#6956=ADVANCED_FACE('',(#1077),#149,.F.);
#6957=ADVANCED_FACE('',(#1078),#150,.F.);
#6958=ADVANCED_FACE('',(#1079),#151,.F.);
#6959=ADVANCED_FACE('',(#1080),#152,.F.);
#6960=ADVANCED_FACE('',(#1081),#153,.F.);
#6961=ADVANCED_FACE('',(#1082),#786,.F.);
#6962=ADVANCED_FACE('',(#1083,#636,#637,#638,#639,#640,#641),#787,.T.);
#6963=ADVANCED_FACE('',(#1084),#154,.F.);
#6964=ADVANCED_FACE('',(#1085),#788,.F.);
#7108=CLOSED_SHELL('',(#6866,#6867,#6868,#6869,#6870,#6871,#6872,#6873,
#6874,#6875,#6876,#6877,#6878,#6879,#6880,#6881,#6882,#6883,#6884,#6885,
#6886,#6887,#6888,#6889,#6890,#6891,#6892,#6893,#6894,#6895,#6896,#6897,
#6898,#6899,#6900,#6901,#6902,#6903,#6904,#6905,#6906,#6907,#6908,#6909,
#6910,#6911,#6912,#6913,#6914,#6915,#6916,#6917,#6918,#6919,#6920,#6921,
#6922,#6923,#6924,#6925,#6926,#6927,#6928,#6929,#6930,#6931,#6932,#6933,
#6934,#6935,#6936,#6937,#6938,#6939,#6940,#6941,#6942,#6943,#6944,#6945,
#6946,#6947,#6948,#6949,#6950,#6951,#6952,#6953,#6954,#6955,#6956,#6957,
#6958,#6959,#6960,#6961,#6962,#6963,#6964));
#7475=AXIS2_PLACEMENT_3D('',#11769,#8484,#8485);
#7476=AXIS2_PLACEMENT_3D('',#11770,#8486,#8487);
#7477=AXIS2_PLACEMENT_3D('',#11836,#8490,#8491);
#7478=AXIS2_PLACEMENT_3D('',#11838,#8492,#8493);
#7479=AXIS2_PLACEMENT_3D('',#11840,#8494,#8495);
#7480=AXIS2_PLACEMENT_3D('',#11841,#8496,#8497);
#7481=AXIS2_PLACEMENT_3D('',#11843,#8498,#8499);
#7482=AXIS2_PLACEMENT_3D('',#11846,#8501,#8502);
#7483=AXIS2_PLACEMENT_3D('',#11847,#8503,#8504);
#7484=AXIS2_PLACEMENT_3D('',#11849,#8505,#8506);
#7485=AXIS2_PLACEMENT_3D('',#11851,#8508,#8509);
#7486=AXIS2_PLACEMENT_3D('',#11853,#8510,#8511);
#7487=AXIS2_PLACEMENT_3D('',#11855,#8513,#8514);
#7488=AXIS2_PLACEMENT_3D('',#11857,#8515,#8516);
#7489=AXIS2_PLACEMENT_3D('',#11860,#8518,#8519);
#7490=AXIS2_PLACEMENT_3D('',#11861,#8520,#8521);
#7491=AXIS2_PLACEMENT_3D('',#11870,#8526,#8527);
#7492=AXIS2_PLACEMENT_3D('',#11876,#8531,#8532);
#7493=AXIS2_PLACEMENT_3D('',#11882,#8536,#8537);
#7494=AXIS2_PLACEMENT_3D('',#11888,#8541,#8542);
#7495=AXIS2_PLACEMENT_3D('',#11894,#8546,#8547);
#7496=AXIS2_PLACEMENT_3D('',#11897,#8550,#8551);
#7497=AXIS2_PLACEMENT_3D('',#11899,#8552,#8553);
#7498=AXIS2_PLACEMENT_3D('',#11900,#8554,#8555);
#7499=AXIS2_PLACEMENT_3D('',#11909,#8560,#8561);
#7500=AXIS2_PLACEMENT_3D('',#11915,#8565,#8566);
#7501=AXIS2_PLACEMENT_3D('',#11921,#8570,#8571);
#7502=AXIS2_PLACEMENT_3D('',#11927,#8575,#8576);
#7503=AXIS2_PLACEMENT_3D('',#11933,#8580,#8581);
#7504=AXIS2_PLACEMENT_3D('',#11936,#8584,#8585);
#7505=AXIS2_PLACEMENT_3D('',#11938,#8586,#8587);
#7506=AXIS2_PLACEMENT_3D('',#11939,#8588,#8589);
#7507=AXIS2_PLACEMENT_3D('',#11942,#8591,#8592);
#7508=AXIS2_PLACEMENT_3D('',#11943,#8593,#8594);
#7509=AXIS2_PLACEMENT_3D('',#11946,#8596,#8597);
#7510=AXIS2_PLACEMENT_3D('',#11947,#8598,#8599);
#7511=AXIS2_PLACEMENT_3D('',#11956,#8604,#8605);
#7512=AXIS2_PLACEMENT_3D('',#11965,#8610,#8611);
#7513=AXIS2_PLACEMENT_3D('',#11974,#8616,#8617);
#7514=AXIS2_PLACEMENT_3D('',#11983,#8622,#8623);
#7515=AXIS2_PLACEMENT_3D('',#11992,#8628,#8629);
#7516=AXIS2_PLACEMENT_3D('',#12001,#8634,#8635);
#7517=AXIS2_PLACEMENT_3D('',#12010,#8640,#8641);
#7518=AXIS2_PLACEMENT_3D('',#12012,#8642,#8643);
#7519=AXIS2_PLACEMENT_3D('',#12013,#8644,#8645);
#7520=AXIS2_PLACEMENT_3D('',#12015,#8646,#8647);
#7521=AXIS2_PLACEMENT_3D('',#12016,#8648,#8649);
#7522=AXIS2_PLACEMENT_3D('',#12019,#8652,#8653);
#7523=AXIS2_PLACEMENT_3D('',#12022,#8656,#8657);
#7524=AXIS2_PLACEMENT_3D('',#12025,#8660,#8661);
#7525=AXIS2_PLACEMENT_3D('',#12031,#8665,#8666);
#7526=AXIS2_PLACEMENT_3D('',#12037,#8670,#8671);
#7527=AXIS2_PLACEMENT_3D('',#12114,#8674,#8675);
#7528=AXIS2_PLACEMENT_3D('',#12192,#8679,#8680);
#7529=AXIS2_PLACEMENT_3D('',#12270,#8684,#8685);
#7530=AXIS2_PLACEMENT_3D('',#12345,#8688,#8689);
#7531=AXIS2_PLACEMENT_3D('',#12361,#8693,#8694);
#7532=AXIS2_PLACEMENT_3D('',#12739,#8706,#8707);
#7533=AXIS2_PLACEMENT_3D('',#12741,#8708,#8709);
#7534=AXIS2_PLACEMENT_3D('',#12743,#8711,#8712);
#7535=AXIS2_PLACEMENT_3D('',#12745,#8714,#8715);
#7536=AXIS2_PLACEMENT_3D('',#12913,#8717,#8718);
#7537=AXIS2_PLACEMENT_3D('',#12914,#8719,#8720);
#7538=AXIS2_PLACEMENT_3D('',#12919,#8721,#8722);
#7539=AXIS2_PLACEMENT_3D('',#12991,#8724,#8725);
#7540=AXIS2_PLACEMENT_3D('',#13109,#8727,#8728);
#7541=AXIS2_PLACEMENT_3D('',#13154,#8729,#8730);
#7542=AXIS2_PLACEMENT_3D('',#13305,#8731,#8732);
#7543=AXIS2_PLACEMENT_3D('',#13425,#8734,#8735);
#7544=AXIS2_PLACEMENT_3D('',#13430,#8736,#8737);
#7545=AXIS2_PLACEMENT_3D('',#13482,#8739,#8740);
#7546=AXIS2_PLACEMENT_3D('',#13483,#8741,#8742);
#7547=AXIS2_PLACEMENT_3D('',#13484,#8743,#8744);
#7548=AXIS2_PLACEMENT_3D('',#13485,#8745,#8746);
#7549=AXIS2_PLACEMENT_3D('',#13486,#8747,#8748);
#7550=AXIS2_PLACEMENT_3D('',#13487,#8749,#8750);
#7551=AXIS2_PLACEMENT_3D('',#13489,#8751,#8752);
#7552=AXIS2_PLACEMENT_3D('',#13490,#8753,#8754);
#7553=AXIS2_PLACEMENT_3D('',#13491,#8755,#8756);
#7554=AXIS2_PLACEMENT_3D('',#13492,#8757,#8758);
#7555=AXIS2_PLACEMENT_3D('',#13493,#8759,#8760);
#7556=AXIS2_PLACEMENT_3D('',#13494,#8761,#8762);
#7557=AXIS2_PLACEMENT_3D('',#13515,#8763,#8764);
#7558=AXIS2_PLACEMENT_3D('',#13517,#8765,#8766);
#7559=AXIS2_PLACEMENT_3D('',#13518,#8767,#8768);
#7560=AXIS2_PLACEMENT_3D('',#13519,#8769,#8770);
#7561=AXIS2_PLACEMENT_3D('',#13617,#8772,#8773);
#7562=AXIS2_PLACEMENT_3D('',#13618,#8774,#8775);
#7563=AXIS2_PLACEMENT_3D('',#13621,#8776,#8777);
#7564=AXIS2_PLACEMENT_3D('',#13623,#8778,#8779);
#7565=AXIS2_PLACEMENT_3D('',#13624,#8780,#8781);
#7566=AXIS2_PLACEMENT_3D('',#13625,#8782,#8783);
#7567=AXIS2_PLACEMENT_3D('',#13628,#8784,#8785);
#7568=AXIS2_PLACEMENT_3D('',#13630,#8786,#8787);
#7569=AXIS2_PLACEMENT_3D('',#13631,#8788,#8789);
#7570=AXIS2_PLACEMENT_3D('',#13632,#8790,#8791);
#7571=AXIS2_PLACEMENT_3D('',#13635,#8792,#8793);
#7572=AXIS2_PLACEMENT_3D('',#13637,#8794,#8795);
#7573=AXIS2_PLACEMENT_3D('',#13638,#8796,#8797);
#7574=AXIS2_PLACEMENT_3D('',#13639,#8798,#8799);
#7575=AXIS2_PLACEMENT_3D('',#13670,#8802,#8803);
#7576=AXIS2_PLACEMENT_3D('',#13673,#8804,#8805);
#7577=AXIS2_PLACEMENT_3D('',#13675,#8806,#8807);
#7578=AXIS2_PLACEMENT_3D('',#13676,#8808,#8809);
#7579=AXIS2_PLACEMENT_3D('',#13677,#8810,#8811);
#7580=AXIS2_PLACEMENT_3D('',#13858,#8814,#8815);
#7581=AXIS2_PLACEMENT_3D('',#13859,#8816,#8817);
#7582=AXIS2_PLACEMENT_3D('',#13876,#8818,#8819);
#8484=DIRECTION('axis',(0.,0.,1.));
#8485=DIRECTION('refdir',(1.,0.,0.));
#8486=DIRECTION('center_axis',(-9.61618982193066E-33,1.03600583455278E-18,
1.));
#8487=DIRECTION('ref_axis',(1.,0.,9.61618982193066E-33));
#8488=DIRECTION('',(0.,-1.,1.03600583455278E-18));
#8489=DIRECTION('',(0.,1.,-1.03600583455278E-18));
#8490=DIRECTION('center_axis',(-9.61618982193066E-33,1.03600583455278E-18,
1.));
#8491=DIRECTION('ref_axis',(1.,0.,0.));
#8492=DIRECTION('center_axis',(-9.61618982193066E-33,1.03600583455278E-18,
1.));
#8493=DIRECTION('ref_axis',(1.,0.,0.));
#8494=DIRECTION('center_axis',(-9.61618982193066E-33,1.03600583455278E-18,
1.));
#8495=DIRECTION('ref_axis',(1.,0.,0.));
#8496=DIRECTION('center_axis',(0.,0.,-1.));
#8497=DIRECTION('ref_axis',(1.,0.,0.));
#8498=DIRECTION('center_axis',(9.61618982193066E-33,-1.03600583455278E-18,
-1.));
#8499=DIRECTION('ref_axis',(1.,0.,0.));
#8500=DIRECTION('',(0.,0.,-1.));
#8501=DIRECTION('center_axis',(-9.61618982193066E-33,1.03600583455278E-18,
1.));
#8502=DIRECTION('ref_axis',(1.,0.,0.));
#8503=DIRECTION('center_axis',(0.,0.,-1.));
#8504=DIRECTION('ref_axis',(1.,0.,0.));
#8505=DIRECTION('center_axis',(9.61618982193066E-33,-1.03600583455278E-18,
-1.));
#8506=DIRECTION('ref_axis',(1.,0.,0.));
#8507=DIRECTION('',(0.,0.,-1.));
#8508=DIRECTION('center_axis',(0.,0.,-1.));
#8509=DIRECTION('ref_axis',(1.,0.,0.));
#8510=DIRECTION('center_axis',(9.61618982193066E-33,-1.03600583455278E-18,
-1.));
#8511=DIRECTION('ref_axis',(1.,0.,0.));
#8512=DIRECTION('',(0.,0.,-1.));
#8513=DIRECTION('center_axis',(0.,0.,-1.));
#8514=DIRECTION('ref_axis',(1.,0.,0.));
#8515=DIRECTION('center_axis',(9.61618982193066E-33,-1.03600583455278E-18,
-1.));
#8516=DIRECTION('ref_axis',(1.,0.,0.));
#8517=DIRECTION('',(0.,0.,-1.));
#8518=DIRECTION('center_axis',(-9.61618982193066E-33,1.03600583455278E-18,
1.));
#8519=DIRECTION('ref_axis',(1.,0.,0.));
#8520=DIRECTION('center_axis',(0.86602540378444,0.499999999999998,0.));
#8521=DIRECTION('ref_axis',(0.499999999999998,-0.86602540378444,0.));
#8522=DIRECTION('',(0.499999999999998,-0.86602540378444,8.9720737119161E-19));
#8523=DIRECTION('',(0.,0.,-1.));
#8524=DIRECTION('',(0.499999999999998,-0.86602540378444,0.));
#8525=DIRECTION('',(0.,0.,-1.));
#8526=DIRECTION('center_axis',(1.60246890531964E-16,1.,0.));
#8527=DIRECTION('ref_axis',(1.,-1.60246890531964E-16,0.));
#8528=DIRECTION('',(1.,-1.60246890531964E-16,9.78220653549071E-33));
#8529=DIRECTION('',(0.,0.,-1.));
#8530=DIRECTION('',(1.,-1.60246890531964E-16,0.));
#8531=DIRECTION('center_axis',(-0.86602540378444,0.499999999999998,0.));
#8532=DIRECTION('ref_axis',(0.499999999999998,0.86602540378444,0.));
#8533=DIRECTION('',(0.499999999999998,0.86602540378444,-8.97207371191601E-19));
#8534=DIRECTION('',(0.,0.,-1.));
#8535=DIRECTION('',(0.499999999999998,0.86602540378444,0.));
#8536=DIRECTION('center_axis',(-0.86602540378444,-0.499999999999998,0.));
#8537=DIRECTION('ref_axis',(-0.499999999999998,0.86602540378444,0.));
#8538=DIRECTION('',(-0.499999999999998,0.86602540378444,-8.9720737119161E-19));
#8539=DIRECTION('',(0.,0.,-1.));
#8540=DIRECTION('',(-0.499999999999998,0.86602540378444,0.));
#8541=DIRECTION('center_axis',(-1.60246890531964E-16,-1.,0.));
#8542=DIRECTION('ref_axis',(-1.,1.60246890531964E-16,0.));
#8543=DIRECTION('',(-1.,1.60246890531964E-16,-9.78220653549071E-33));
#8544=DIRECTION('',(0.,0.,-1.));
#8545=DIRECTION('',(-1.,1.60246890531964E-16,0.));
#8546=DIRECTION('center_axis',(0.86602540378444,-0.499999999999998,0.));
#8547=DIRECTION('ref_axis',(-0.499999999999998,-0.86602540378444,0.));
#8548=DIRECTION('',(-0.499999999999998,-0.86602540378444,8.97207371191601E-19));
#8549=DIRECTION('',(-0.499999999999998,-0.86602540378444,0.));
#8550=DIRECTION('center_axis',(0.,0.,-1.));
#8551=DIRECTION('ref_axis',(-1.,0.,0.));
#8552=DIRECTION('center_axis',(0.,0.,1.));
#8553=DIRECTION('ref_axis',(1.,0.,0.));
#8554=DIRECTION('center_axis',(0.866025403784439,0.5,0.));
#8555=DIRECTION('ref_axis',(0.5,-0.866025403784439,0.));
#8556=DIRECTION('',(0.5,-0.866025403784439,8.97207371191609E-19));
#8557=DIRECTION('',(0.,0.,-1.));
#8558=DIRECTION('',(0.5,-0.866025403784439,0.));
#8559=DIRECTION('',(0.,0.,-1.));
#8560=DIRECTION('center_axis',(1.60246890531964E-16,1.,0.));
#8561=DIRECTION('ref_axis',(1.,-1.60246890531964E-16,0.));
#8562=DIRECTION('',(1.,-1.60246890531964E-16,9.78220653549071E-33));
#8563=DIRECTION('',(0.,0.,-1.));
#8564=DIRECTION('',(1.,-1.60246890531964E-16,0.));
#8565=DIRECTION('center_axis',(-0.866025403784438,0.5,0.));
#8566=DIRECTION('ref_axis',(0.5,0.866025403784438,0.));
#8567=DIRECTION('',(0.5,0.866025403784438,-8.97207371191599E-19));
#8568=DIRECTION('',(0.,0.,-1.));
#8569=DIRECTION('',(0.5,0.866025403784438,0.));
#8570=DIRECTION('center_axis',(-0.866025403784439,-0.499999999999999,0.));
#8571=DIRECTION('ref_axis',(-0.499999999999999,0.866025403784439,0.));
#8572=DIRECTION('',(-0.499999999999999,0.866025403784439,-8.97207371191609E-19));
#8573=DIRECTION('',(0.,0.,-1.));
#8574=DIRECTION('',(-0.499999999999999,0.866025403784439,0.));
#8575=DIRECTION('center_axis',(-1.60246890531964E-16,-1.,0.));
#8576=DIRECTION('ref_axis',(-1.,1.60246890531964E-16,0.));
#8577=DIRECTION('',(-1.,1.60246890531964E-16,-9.78220653549071E-33));
#8578=DIRECTION('',(0.,0.,-1.));
#8579=DIRECTION('',(-1.,1.60246890531964E-16,0.));
#8580=DIRECTION('center_axis',(0.866025403784439,-0.5,0.));
#8581=DIRECTION('ref_axis',(-0.5,-0.866025403784439,0.));
#8582=DIRECTION('',(-0.5,-0.866025403784439,8.97207371191599E-19));
#8583=DIRECTION('',(-0.5,-0.866025403784439,0.));
#8584=DIRECTION('center_axis',(0.,0.,-1.));
#8585=DIRECTION('ref_axis',(-1.,0.,0.));
#8586=DIRECTION('center_axis',(0.,0.,1.));
#8587=DIRECTION('ref_axis',(1.,0.,0.));
#8588=DIRECTION('center_axis',(0.,0.,-1.));
#8589=DIRECTION('ref_axis',(1.,0.,0.));
#8590=DIRECTION('',(0.,0.,-1.));
#8591=DIRECTION('center_axis',(0.,0.,1.));
#8592=DIRECTION('ref_axis',(1.,0.,0.));
#8593=DIRECTION('center_axis',(0.,0.,-1.));
#8594=DIRECTION('ref_axis',(1.,0.,0.));
#8595=DIRECTION('',(0.,0.,-1.));
#8596=DIRECTION('center_axis',(0.,0.,1.));
#8597=DIRECTION('ref_axis',(1.,0.,0.));
#8598=DIRECTION('center_axis',(0.,-1.,0.));
#8599=DIRECTION('ref_axis',(-1.,0.,0.));
#8600=DIRECTION('',(0.0523359562429438,0.,0.998629534754574));
#8601=DIRECTION('',(1.,0.,0.));
#8602=DIRECTION('',(-0.0523359562429438,0.,-0.998629534754574));
#8603=DIRECTION('',(1.,0.,0.));
#8604=DIRECTION('center_axis',(0.,-1.,0.));
#8605=DIRECTION('ref_axis',(-1.,0.,0.));
#8606=DIRECTION('',(0.,0.,-1.));
#8607=DIRECTION('',(1.,0.,0.));
#8608=DIRECTION('',(0.,0.,1.));
#8609=DIRECTION('',(1.,0.,0.));
#8610=DIRECTION('center_axis',(0.,-1.,0.));
#8611=DIRECTION('ref_axis',(-1.,0.,0.));
#8612=DIRECTION('',(0.,0.,-1.));
#8613=DIRECTION('',(1.,0.,0.));
#8614=DIRECTION('',(0.,0.,1.));
#8615=DIRECTION('',(1.,0.,0.));
#8616=DIRECTION('center_axis',(0.,-1.,0.));
#8617=DIRECTION('ref_axis',(-1.,0.,0.));
#8618=DIRECTION('',(0.,0.,-1.));
#8619=DIRECTION('',(1.,0.,0.));
#8620=DIRECTION('',(0.,0.,1.));
#8621=DIRECTION('',(1.,0.,0.));
#8622=DIRECTION('center_axis',(0.,1.,0.));
#8623=DIRECTION('ref_axis',(1.,0.,0.));
#8624=DIRECTION('',(-0.0523359562429438,0.,-0.998629534754574));
#8625=DIRECTION('',(-1.,0.,0.));
#8626=DIRECTION('',(0.0523359562429438,0.,0.998629534754574));
#8627=DIRECTION('',(-1.,0.,0.));
#8628=DIRECTION('center_axis',(0.,1.,0.));
#8629=DIRECTION('ref_axis',(1.,0.,0.));
#8630=DIRECTION('',(0.,0.,1.));
#8631=DIRECTION('',(-1.,0.,0.));
#8632=DIRECTION('',(0.,0.,-1.));
#8633=DIRECTION('',(-1.,0.,0.));
#8634=DIRECTION('center_axis',(0.,1.,0.));
#8635=DIRECTION('ref_axis',(1.,0.,0.));
#8636=DIRECTION('',(0.,0.,1.));
#8637=DIRECTION('',(-1.,0.,0.));
#8638=DIRECTION('',(0.,0.,-1.));
#8639=DIRECTION('',(-1.,0.,0.));
#8640=DIRECTION('center_axis',(0.,0.,1.));
#8641=DIRECTION('ref_axis',(1.,0.,0.));
#8642=DIRECTION('center_axis',(0.,0.,1.));
#8643=DIRECTION('ref_axis',(1.,0.,0.));
#8644=DIRECTION('center_axis',(0.,0.,1.));
#8645=DIRECTION('ref_axis',(1.,0.,0.));
#8646=DIRECTION('center_axis',(0.,0.,1.));
#8647=DIRECTION('ref_axis',(1.,0.,0.));
#8648=DIRECTION('center_axis',(0.,0.,1.));
#8649=DIRECTION('ref_axis',(1.,0.,0.));
#8650=DIRECTION('',(0.,1.,0.));
#8651=DIRECTION('',(0.,-1.,0.));
#8652=DIRECTION('center_axis',(0.,0.,1.));
#8653=DIRECTION('ref_axis',(1.,0.,0.));
#8654=DIRECTION('',(0.,-1.,0.));
#8655=DIRECTION('',(0.,1.,0.));
#8656=DIRECTION('center_axis',(0.,0.,1.));
#8657=DIRECTION('ref_axis',(1.,0.,0.));
#8658=DIRECTION('',(0.,-1.,0.));
#8659=DIRECTION('',(0.,1.,0.));
#8660=DIRECTION('center_axis',(0.,0.,1.));
#8661=DIRECTION('ref_axis',(1.,0.,0.));
#8662=DIRECTION('',(0.,-1.,0.));
#8663=DIRECTION('',(-1.,0.,0.));
#8664=DIRECTION('',(0.,1.,0.));
#8665=DIRECTION('center_axis',(0.,1.,0.));
#8666=DIRECTION('ref_axis',(1.,0.,0.));
#8667=DIRECTION('',(0.,0.,1.));
#8668=DIRECTION('',(-1.,0.,0.));
#8669=DIRECTION('',(0.,0.,-1.));
#8670=DIRECTION('center_axis',(-1.,0.,0.));
#8671=DIRECTION('ref_axis',(0.,-1.,0.));
#8672=DIRECTION('',(0.,-1.,0.));
#8673=DIRECTION('',(0.,-1.,1.03600583455278E-18));
#8674=DIRECTION('center_axis',(1.,0.,0.));
#8675=DIRECTION('ref_axis',(0.,1.,0.));
#8676=DIRECTION('',(0.,1.,0.));
#8677=DIRECTION('',(0.,1.,-1.03600583455278E-18));
#8678=DIRECTION('',(0.,1.,0.));
#8679=DIRECTION('center_axis',(1.,0.,0.));
#8680=DIRECTION('ref_axis',(0.,1.,0.));
#8681=DIRECTION('',(0.,1.,0.));
#8682=DIRECTION('',(0.,1.,-1.03600583455278E-18));
#8683=DIRECTION('',(0.,1.,0.));
#8684=DIRECTION('center_axis',(1.,0.,0.));
#8685=DIRECTION('ref_axis',(0.,1.,0.));
#8686=DIRECTION('',(0.,1.,0.));
#8687=DIRECTION('',(0.,1.,0.));
#8688=DIRECTION('center_axis',(0.998629534754574,0.,-0.0523359562429438));
#8689=DIRECTION('ref_axis',(-0.0523359562429438,0.,-0.998629534754574));
#8690=DIRECTION('',(0.,-1.,0.));
#8691=DIRECTION('',(5.42947651131849E-20,-1.,1.03600583455278E-18));
#8692=DIRECTION('',(0.,-1.,0.));
#8693=DIRECTION('center_axis',(0.,0.,1.));
#8694=DIRECTION('ref_axis',(1.,0.,0.));
#8695=DIRECTION('',(0.,-1.,0.));
#8696=DIRECTION('',(0.,-1.,0.));
#8697=DIRECTION('',(0.,-1.,0.));
#8698=DIRECTION('',(0.,1.,0.));
#8699=DIRECTION('',(0.,-1.,0.));
#8700=DIRECTION('',(0.,1.,0.));
#8701=DIRECTION('',(0.,-1.,0.));
#8702=DIRECTION('',(0.,-1.,0.));
#8703=DIRECTION('',(0.,-1.,0.));
#8704=DIRECTION('',(0.,1.,0.));
#8705=DIRECTION('',(0.,1.,0.));
#8706=DIRECTION('center_axis',(0.,0.,1.));
#8707=DIRECTION('ref_axis',(1.,0.,0.));
#8708=DIRECTION('center_axis',(-9.61618982193066E-33,1.03600583455278E-18,
1.));
#8709=DIRECTION('ref_axis',(1.,0.,0.));
#8710=DIRECTION('',(0.,0.,-1.));
#8711=DIRECTION('center_axis',(0.,0.,1.));
#8712=DIRECTION('ref_axis',(1.,0.,0.));
#8713=DIRECTION('',(0.,0.,-1.));
#8714=DIRECTION('center_axis',(1.,0.,0.));
#8715=DIRECTION('ref_axis',(0.,1.,0.));
#8716=DIRECTION('',(0.,1.,-1.03600583455278E-18));
#8717=DIRECTION('center_axis',(0.994044372876412,-0.108976074221552,-1.1933167131821E-14));
#8718=DIRECTION('ref_axis',(-0.108857570442347,-0.992963419871597,0.0466226999892957));
#8719=DIRECTION('center_axis',(-9.61618982193066E-33,1.03600583455278E-18,
1.));
#8720=DIRECTION('ref_axis',(1.,0.,9.61618982193066E-33));
#8721=DIRECTION('center_axis',(-9.61618982193066E-33,1.03600583455278E-18,
1.));
#8722=DIRECTION('ref_axis',(1.,0.,9.61618982193066E-33));
#8723=DIRECTION('',(-5.42947651131849E-20,-1.,1.03600583455278E-18));
#8724=DIRECTION('center_axis',(-1.,0.,0.));
#8725=DIRECTION('ref_axis',(0.,-1.,0.));
#8726=DIRECTION('',(0.,-1.,1.03600583455278E-18));
#8727=DIRECTION('center_axis',(-9.61618982193066E-33,1.03600583455278E-18,
1.));
#8728=DIRECTION('ref_axis',(1.,0.,9.61618982193066E-33));
#8729=DIRECTION('center_axis',(-1.,0.,0.));
#8730=DIRECTION('ref_axis',(0.,-1.,0.));
#8731=DIRECTION('center_axis',(-1.,0.,0.));
#8732=DIRECTION('ref_axis',(0.,-1.,0.));
#8733=DIRECTION('',(0.,-1.,1.03600583455278E-18));
#8734=DIRECTION('center_axis',(-0.999738255753194,0.0228783737088345,0.));
#8735=DIRECTION('ref_axis',(0.,0.,1.));
#8736=DIRECTION('center_axis',(-9.61618982193066E-33,1.03600583455278E-18,
1.));
#8737=DIRECTION('ref_axis',(1.,0.,9.61618982193066E-33));
#8738=DIRECTION('',(-5.42947651131849E-20,1.,-1.03600583455278E-18));
#8739=DIRECTION('center_axis',(-0.999738255790058,-0.0228783720979604,1.69987959829136E-9));
#8740=DIRECTION('ref_axis',(-0.022845652001536,0.998308458201847,0.0534630570326489));
#8741=DIRECTION('center_axis',(-0.375013085256251,-0.833398400631247,0.405970801550885));
#8742=DIRECTION('ref_axis',(-0.565498005067694,0.552672693214782,0.612180447612612));
#8743=DIRECTION('center_axis',(-7.78474640228738E-11,1.,0.));
#8744=DIRECTION('ref_axis',(0.,0.,1.));
#8745=DIRECTION('center_axis',(0.0522645732252412,-0.0522112666801462,0.997267465636596));
#8746=DIRECTION('ref_axis',(-0.998629534754574,0.,0.0523359562429445));
#8747=DIRECTION('center_axis',(0.361627795167438,-0.818371417997736,0.44664701943113));
#8748=DIRECTION('ref_axis',(0.514966362801186,0.574689674697898,0.636035708886648));
#8749=DIRECTION('center_axis',(0.994044372876412,0.108976074221546,-5.96658356591051E-15));
#8750=DIRECTION('ref_axis',(5.9211894646675E-15,7.40148683083438E-16,1.));
#8751=DIRECTION('center_axis',(-0.052263633556273,-0.0525535553916586,0.997249535684621));
#8752=DIRECTION('ref_axis',(-0.108857570442347,0.992963419871597,0.0466226999892949));
#8753=DIRECTION('center_axis',(0.,1.,0.));
#8754=DIRECTION('ref_axis',(0.998629534754574,0.,0.0523359562429438));
#8755=DIRECTION('center_axis',(0.375013085403515,-0.833398400816333,-0.405970801034895));
#8756=DIRECTION('ref_axis',(-0.565498005700927,-0.552672692935682,0.612180447279637));
#8757=DIRECTION('center_axis',(0.0522645732252408,0.0522112666801459,0.997267465636596));
#8758=DIRECTION('ref_axis',(-0.0228456520015352,-0.998308458201847,0.0534630570326489));
#8759=DIRECTION('center_axis',(-4.07418268117644E-12,-1.,-7.77400366303027E-11));
#8760=DIRECTION('ref_axis',(-0.998629534754574,0.,0.0523359562429438));
#8761=DIRECTION('center_axis',(-5.42947651131849E-20,1.,-1.03600583455278E-18));
#8762=DIRECTION('ref_axis',(-0.688354575693754,0.,0.725374371012288));
#8763=DIRECTION('center_axis',(-0.361627795167436,-0.818371417997736,-0.446647019431131));
#8764=DIRECTION('ref_axis',(0.514966362801185,-0.574689674697896,0.636035708886651));
#8765=DIRECTION('center_axis',(-0.0522636335562752,0.0525535553916633,0.99724953568462));
#8766=DIRECTION('ref_axis',(0.998629534754574,0.,0.0523359562429442));
#8767=DIRECTION('center_axis',(0.,-1.,0.));
#8768=DIRECTION('ref_axis',(0.,0.,1.));
#8769=DIRECTION('center_axis',(-5.42947651131849E-20,-1.,1.03600583455278E-18));
#8770=DIRECTION('ref_axis',(0.688354575693754,0.,0.725374371012288));
#8771=DIRECTION('',(5.42947651131849E-20,1.,-1.03600583455278E-18));
#8772=DIRECTION('center_axis',(-0.998629534754574,0.,-0.0523359562429438));
#8773=DIRECTION('ref_axis',(-0.0523359562429438,0.,0.998629534754574));
#8774=DIRECTION('center_axis',(-0.375013085256251,-0.833398400631247,0.405970801550885));
#8775=DIRECTION('ref_axis',(-0.565498005067695,0.552672693214781,0.612180447612612));
#8776=DIRECTION('center_axis',(-7.78474640228738E-11,1.,0.));
#8777=DIRECTION('ref_axis',(0.,0.,1.));
#8778=DIRECTION('center_axis',(-0.999738255790058,-0.0228783720979604,1.69987959829136E-9));
#8779=DIRECTION('ref_axis',(-0.022845652001536,0.998308458201847,0.0534630570326489));
#8780=DIRECTION('center_axis',(0.0522645732252412,-0.0522112666801462,0.997267465636596));
#8781=DIRECTION('ref_axis',(-0.998629534754574,0.,0.0523359562429445));
#8782=DIRECTION('center_axis',(0.361627795167442,-0.818371417997735,0.446647019431129));
#8783=DIRECTION('ref_axis',(0.514966362801186,0.574689674697898,0.636035708886649));
#8784=DIRECTION('center_axis',(0.994044372876412,0.108976074221546,-5.96658356591051E-15));
#8785=DIRECTION('ref_axis',(5.9211894646675E-15,7.40148683083438E-16,1.));
#8786=DIRECTION('center_axis',(0.,1.,0.));
#8787=DIRECTION('ref_axis',(0.998629534754574,0.,0.0523359562429438));
#8788=DIRECTION('center_axis',(-0.052263633556273,-0.0525535553916586,0.997249535684621));
#8789=DIRECTION('ref_axis',(-0.108857570442347,0.992963419871597,0.0466226999892949));
#8790=DIRECTION('center_axis',(0.375013085403515,-0.833398400816333,-0.405970801034895));
#8791=DIRECTION('ref_axis',(-0.565498005700926,-0.552672692935682,0.612180447279637));
#8792=DIRECTION('center_axis',(-0.999738255753194,0.0228783737088345,0.));
#8793=DIRECTION('ref_axis',(0.,0.,1.));
#8794=DIRECTION('center_axis',(-4.07418268117644E-12,-1.,-7.77400366303027E-11));
#8795=DIRECTION('ref_axis',(-0.998629534754574,0.,0.0523359562429438));
#8796=DIRECTION('center_axis',(0.0522645732252408,0.0522112666801459,0.997267465636596));
#8797=DIRECTION('ref_axis',(-0.0228456520015352,-0.998308458201847,0.0534630570326489));
#8798=DIRECTION('center_axis',(-5.42947651131849E-20,1.,-1.03600583455278E-18));
#8799=DIRECTION('ref_axis',(-0.688354575693754,0.,0.725374371012288));
#8800=DIRECTION('',(5.42947651131849E-20,-1.,1.03600583455278E-18));
#8801=DIRECTION('',(-5.42947651131849E-20,1.,-1.03600583455278E-18));
#8802=DIRECTION('center_axis',(-0.361627795167436,-0.818371417997736,-0.446647019431131));
#8803=DIRECTION('ref_axis',(0.51496636280118,-0.574689674697898,0.636035708886653));
#8804=DIRECTION('center_axis',(-0.0522636335562752,0.0525535553916633,0.99724953568462));
#8805=DIRECTION('ref_axis',(0.998629534754574,0.,0.0523359562429441));
#8806=DIRECTION('center_axis',(0.,-1.,0.));
#8807=DIRECTION('ref_axis',(0.,0.,1.));
#8808=DIRECTION('center_axis',(0.994044372876412,-0.108976074221552,-1.1933167131821E-14));
#8809=DIRECTION('ref_axis',(-0.108857570442347,-0.992963419871597,0.0466226999892957));
#8810=DIRECTION('center_axis',(-5.42947651131849E-20,-1.,1.03600583455278E-18));
#8811=DIRECTION('ref_axis',(0.688354575693754,0.,0.725374371012288));
#8812=DIRECTION('',(5.42947651131849E-20,1.,-1.03600583455278E-18));
#8813=DIRECTION('',(-5.42947651131849E-20,-1.,1.03600583455278E-18));
#8814=DIRECTION('center_axis',(0.998629534754574,0.,-0.0523359562429438));
#8815=DIRECTION('ref_axis',(-0.0523359562429438,0.,-0.998629534754574));
#8816=DIRECTION('center_axis',(-9.61618982193066E-33,1.03600583455278E-18,
1.));
#8817=DIRECTION('ref_axis',(1.,0.,9.61618982193066E-33));
#8818=DIRECTION('center_axis',(-0.998629534754574,0.,-0.0523359562429438));
#8819=DIRECTION('ref_axis',(-0.0523359562429438,0.,0.998629534754574));
#11769=CARTESIAN_POINT('',(0.,0.,0.));
#11770=CARTESIAN_POINT('Origin',(6.87409734069396,-2.22251806091942E-16,
0.7));
#11771=CARTESIAN_POINT('',(3.31825992066485,1.2493322588334,0.7));
#11772=CARTESIAN_POINT('',(4.3,1.27917501057225,0.7));
#11773=CARTESIAN_POINT('Ctrl Pts',(3.31826243508713,1.24933270901874,0.7));
#11774=CARTESIAN_POINT('Ctrl Pts',(3.64552542112514,1.25866821321074,0.7));
#11775=CARTESIAN_POINT('Ctrl Pts',(3.97277304530853,1.26856018917077,0.7));
#11776=CARTESIAN_POINT('Ctrl Pts',(4.30000000005992,1.27917501058303,0.7));
#11777=CARTESIAN_POINT('',(4.3,-1.27917501057184,0.7));
#11778=CARTESIAN_POINT('',(4.3,0.742407407407408,0.7));
#11779=CARTESIAN_POINT('',(3.31825992075695,-1.24933225883136,0.7));
#11780=CARTESIAN_POINT('Ctrl Pts',(4.3000000000599,-1.27917501058303,0.7));
#11781=CARTESIAN_POINT('Ctrl Pts',(3.97277304533917,-1.26856018917177,0.7));
#11782=CARTESIAN_POINT('Ctrl Pts',(3.64552542118644,-1.25866821321259,0.7));
#11783=CARTESIAN_POINT('Ctrl Pts',(3.3182624351791,-1.24933270902137,0.7));
#11784=CARTESIAN_POINT('',(3.26759951430388,-1.24789152572578,0.7));
#11785=CARTESIAN_POINT('Ctrl Pts',(3.26760216044043,-1.24789199949781,0.7));
#11786=CARTESIAN_POINT('Ctrl Pts',(3.27154046708102,-1.24840675231115,0.699999999449966));
#11787=CARTESIAN_POINT('Ctrl Pts',(3.27549053112987,-1.2488275353013,0.699997549264952));
#11788=CARTESIAN_POINT('Ctrl Pts',(3.27944900419773,-1.24915404112413,0.699995443099811));
#11789=CARTESIAN_POINT('Ctrl Pts',(3.28202272903949,-1.24936632907779,0.699994073710794));
#11790=CARTESIAN_POINT('Ctrl Pts',(3.28459959180148,-1.24953872742098,0.699992815093061));
#11791=CARTESIAN_POINT('Ctrl Pts',(3.28717866899733,-1.24967118132558,0.699992046536556));
#11792=CARTESIAN_POINT('Ctrl Pts',(3.28888409507617,-1.24975876704947,0.699991538325205));
#11793=CARTESIAN_POINT('Ctrl Pts',(3.29059037034979,-1.2498288805585,0.699991238158591));
#11794=CARTESIAN_POINT('Ctrl Pts',(3.29229723346923,-1.24988151179005,0.69999118215758));
#11795=CARTESIAN_POINT('Ctrl Pts',(3.29393274317941,-1.24993194283473,0.699991128497625));
#11796=CARTESIAN_POINT('Ctrl Pts',(3.29556870469678,-1.24996631998408,0.699991298652463));
#11797=CARTESIAN_POINT('Ctrl Pts',(3.29720488848534,-1.24998463806557,0.699991673963628));
#11798=CARTESIAN_POINT('Ctrl Pts',(3.29943508678369,-1.25000960650399,0.699992185531049));
#11799=CARTESIAN_POINT('Ctrl Pts',(3.30166551218918,-1.25000473681137,0.699993084765318));
#11800=CARTESIAN_POINT('Ctrl Pts',(3.30389557412726,-1.24997002667259,0.699994176731177));
#11801=CARTESIAN_POINT('Ctrl Pts',(3.30868977915254,-1.24989540653807,0.699996524248132));
#11802=CARTESIAN_POINT('Ctrl Pts',(3.31348068594496,-1.24968290539118,0.699999999312134));
#11803=CARTESIAN_POINT('Ctrl Pts',(3.3182624351791,-1.24933270902137,0.7));
#11804=CARTESIAN_POINT('',(1.1,-1.19266190204492,0.7));
#11805=CARTESIAN_POINT('Ctrl Pts',(3.26760216044045,-1.24789199949781,0.7));
#11806=CARTESIAN_POINT('Ctrl Pts',(2.54512260523322,-1.2274084473838,0.7));
#11807=CARTESIAN_POINT('Ctrl Pts',(1.82256951666701,-1.20959509718369,0.7));
#11808=CARTESIAN_POINT('Ctrl Pts',(1.09999999999999,-1.19266190204553,0.7));
#11809=CARTESIAN_POINT('',(1.1,1.19266190204492,0.7));
#11810=CARTESIAN_POINT('',(1.1,-0.696450594095222,0.7));
#11811=CARTESIAN_POINT('',(3.26759952419083,1.24789152650872,0.7));
#11812=CARTESIAN_POINT('Ctrl Pts',(1.09999999999999,1.19266190204553,0.7));
#11813=CARTESIAN_POINT('Ctrl Pts',(1.82256951996781,1.20959509726105,0.7));
#11814=CARTESIAN_POINT('Ctrl Pts',(2.54512261183467,1.22740844754655,0.7));
#11815=CARTESIAN_POINT('Ctrl Pts',(3.26760217034162,1.24789199977852,0.7));
#11816=CARTESIAN_POINT('Ctrl Pts',(3.3182624351791,1.24933270902137,0.7));
#11817=CARTESIAN_POINT('Ctrl Pts',(3.3143012451848,1.2496228108833,0.699999999430174));
#11818=CARTESIAN_POINT('Ctrl Pts',(3.31033365565543,1.24981842655856,0.699997549220164));
#11819=CARTESIAN_POINT('Ctrl Pts',(3.30636302717881,1.24991943948955,0.699995443052606));
#11820=CARTESIAN_POINT('Ctrl Pts',(3.30378139908369,1.24998511620097,0.699994073661998));
#11821=CARTESIAN_POINT('Ctrl Pts',(3.3011989045204,1.25001078941611,0.699992815050698));
#11822=CARTESIAN_POINT('Ctrl Pts',(3.29861646861803,1.2499964568765,0.699992046505716));
#11823=CARTESIAN_POINT('Ctrl Pts',(3.2969088217217,1.24998697942277,0.699991538302026));
#11824=CARTESIAN_POINT('Ctrl Pts',(3.29520131971864,1.24996000972381,0.699991238145114));
#11825=CARTESIAN_POINT('Ctrl Pts',(3.29349422410899,1.24991555258537,0.699991182154076));
#11826=CARTESIAN_POINT('Ctrl Pts',(3.29185849176351,1.24987295392896,0.699991128503682));
#11827=CARTESIAN_POINT('Ctrl Pts',(3.29022322047391,1.2498143016413,0.699991298668259));
#11828=CARTESIAN_POINT('Ctrl Pts',(3.28858863969825,1.2497396036024,0.699991673987721));
#11829=CARTESIAN_POINT('Ctrl Pts',(3.286360626573,1.24963778654105,0.699992185566407));
#11830=CARTESIAN_POINT('Ctrl Pts',(3.28413408201674,1.24950616665997,0.699993084809042));
#11831=CARTESIAN_POINT('Ctrl Pts',(3.2819095957713,1.24934477520901,0.699994176777649));
#11832=CARTESIAN_POINT('Ctrl Pts',(3.27712738077041,1.24899781481787,0.699996524298861));
#11833=CARTESIAN_POINT('Ctrl Pts',(3.27235629258357,1.24851338385513,0.699999999330822));
#11834=CARTESIAN_POINT('Ctrl Pts',(3.26760217026193,1.24789200078152,0.699999999999999));
#11835=CARTESIAN_POINT('',(3.15,1.,0.7));
#11836=CARTESIAN_POINT('Origin',(3.3,1.,0.7));
#11837=CARTESIAN_POINT('',(3.15,-1.,0.7));
#11838=CARTESIAN_POINT('Origin',(3.3,-1.,0.7));
#11839=CARTESIAN_POINT('',(1.6,-4.89858719658941E-17,0.7));
#11840=CARTESIAN_POINT('Origin',(2.,0.,0.7));
#11841=CARTESIAN_POINT('Origin',(9.9,-1.,0.8));
#11842=CARTESIAN_POINT('',(9.75,-1.,0.9));
#11843=CARTESIAN_POINT('Origin',(9.9,-1.,0.9));
#11844=CARTESIAN_POINT('',(9.75,-1.,0.7));
#11845=CARTESIAN_POINT('',(9.75,-1.,0.8));
#11846=CARTESIAN_POINT('Origin',(9.9,-1.,0.7));
#11847=CARTESIAN_POINT('Origin',(3.3,-1.,0.8));
#11848=CARTESIAN_POINT('',(3.15,-1.,0.9));
#11849=CARTESIAN_POINT('Origin',(3.3,-1.,0.9));
#11850=CARTESIAN_POINT('',(3.15,-1.,0.8));
#11851=CARTESIAN_POINT('Origin',(3.3,1.,0.8));
#11852=CARTESIAN_POINT('',(3.15,1.,0.9));
#11853=CARTESIAN_POINT('Origin',(3.3,1.,0.9));
#11854=CARTESIAN_POINT('',(3.15,1.,0.8));
#11855=CARTESIAN_POINT('Origin',(9.9,1.,0.8));
#11856=CARTESIAN_POINT('',(9.75,1.,0.9));
#11857=CARTESIAN_POINT('Origin',(9.9,1.,0.9));
#11858=CARTESIAN_POINT('',(9.75,1.,0.7));
#11859=CARTESIAN_POINT('',(9.75,1.,0.8));
#11860=CARTESIAN_POINT('Origin',(9.9,1.,0.7));
#11861=CARTESIAN_POINT('Origin',(11.3732050807569,0.3,0.9));
#11862=CARTESIAN_POINT('',(11.3732050807569,0.3,0.9));
#11863=CARTESIAN_POINT('',(11.5464101615138,0.,0.9));
#11864=CARTESIAN_POINT('',(10.8757685185329,1.16158539931442,0.9));
#11865=CARTESIAN_POINT('',(11.3732050807569,0.3,0.6));
#11866=CARTESIAN_POINT('',(11.3732050807569,0.3,0.9));
#11867=CARTESIAN_POINT('',(11.5464101615138,0.,0.6));
#11868=CARTESIAN_POINT('',(11.5464101615138,0.,0.6));
#11869=CARTESIAN_POINT('',(11.5464101615138,0.,0.9));
#11870=CARTESIAN_POINT('Origin',(11.0267949192431,0.3,0.9));
#11871=CARTESIAN_POINT('',(11.0267949192431,0.3,0.9));
#11872=CARTESIAN_POINT('',(8.95044612996854,0.3,0.9));
#11873=CARTESIAN_POINT('',(11.0267949192431,0.3,0.6));
#11874=CARTESIAN_POINT('',(11.0267949192431,0.3,0.9));
#11875=CARTESIAN_POINT('',(11.3732050807569,0.3,0.6));
#11876=CARTESIAN_POINT('Origin',(10.8535898384862,5.55111512312578E-17,
0.9));
#11877=CARTESIAN_POINT('',(10.8535898384862,4.24230095489963E-17,0.9));
#11878=CARTESIAN_POINT('',(10.3561532762622,-0.86158539931442,0.9));
#11879=CARTESIAN_POINT('',(10.8535898384862,5.55111512312578E-17,0.6));
#11880=CARTESIAN_POINT('',(10.8535898384862,4.24230095489963E-17,0.9));
#11881=CARTESIAN_POINT('',(11.0267949192431,0.3,0.6));
#11882=CARTESIAN_POINT('Origin',(11.0267949192431,-0.3,0.9));
#11883=CARTESIAN_POINT('',(11.0267949192431,-0.3,0.9));
#11884=CARTESIAN_POINT('',(10.4427558166406,0.71158539931442,0.9));
#11885=CARTESIAN_POINT('',(11.0267949192431,-0.3,0.6));
#11886=CARTESIAN_POINT('',(11.0267949192431,-0.3,0.9));
#11887=CARTESIAN_POINT('',(10.8535898384862,4.24230095489963E-17,0.6));
#11888=CARTESIAN_POINT('Origin',(11.3732050807569,-0.3,0.9));
#11889=CARTESIAN_POINT('',(11.3732050807569,-0.3,0.9));
#11890=CARTESIAN_POINT('',(9.12365121072543,-0.3,0.9));
#11891=CARTESIAN_POINT('',(11.3732050807569,-0.3,0.6));
#11892=CARTESIAN_POINT('',(11.3732050807569,-0.3,0.9));
#11893=CARTESIAN_POINT('',(11.0267949192431,-0.3,0.6));
#11894=CARTESIAN_POINT('Origin',(11.5464101615138,0.,0.9));
#11895=CARTESIAN_POINT('',(10.9623710589113,-1.01158539931442,0.9));
#11896=CARTESIAN_POINT('',(11.3732050807569,-0.3,0.6));
#11897=CARTESIAN_POINT('Origin',(11.2,5.55111512312578E-17,0.6));
#11898=CARTESIAN_POINT('',(11.03,-2.0818995585505E-17,0.6));
#11899=CARTESIAN_POINT('Origin',(11.2,0.,0.6));
#11900=CARTESIAN_POINT('Origin',(2.17320508075689,0.3,0.9));
#11901=CARTESIAN_POINT('',(2.17320508075689,0.3,0.9));
#11902=CARTESIAN_POINT('',(2.34641016151378,0.,0.9));
#11903=CARTESIAN_POINT('',(2.82576851853285,-0.830273029389787,0.9));
#11904=CARTESIAN_POINT('',(2.17320508075689,0.3,0.6));
#11905=CARTESIAN_POINT('',(2.17320508075689,0.3,0.9));
#11906=CARTESIAN_POINT('',(2.34641016151378,0.,0.6));
#11907=CARTESIAN_POINT('',(2.34641016151378,0.,0.6));
#11908=CARTESIAN_POINT('',(2.34641016151378,0.,0.9));
#11909=CARTESIAN_POINT('Origin',(1.82679491924311,0.3,0.9));
#11910=CARTESIAN_POINT('',(1.82679491924311,0.3,0.9));
#11911=CARTESIAN_POINT('',(4.35044612996854,0.3,0.9));
#11912=CARTESIAN_POINT('',(1.82679491924311,0.3,0.6));
#11913=CARTESIAN_POINT('',(1.82679491924311,0.3,0.9));
#11914=CARTESIAN_POINT('',(2.17320508075689,0.3,0.6));
#11915=CARTESIAN_POINT('Origin',(1.65358983848622,5.55111512312578E-17,
0.9));
#11916=CARTESIAN_POINT('',(1.65358983848622,4.24230095489963E-17,0.9));
#11917=CARTESIAN_POINT('',(2.30615327626219,1.13027302938979,0.9));
#11918=CARTESIAN_POINT('',(1.65358983848622,5.55111512312578E-17,0.6));
#11919=CARTESIAN_POINT('',(1.65358983848622,4.24230095489963E-17,0.9));
#11920=CARTESIAN_POINT('',(1.82679491924311,0.3,0.6));
#11921=CARTESIAN_POINT('Origin',(1.82679491924311,-0.3,0.9));
#11922=CARTESIAN_POINT('',(1.82679491924311,-0.3,0.9));
#11923=CARTESIAN_POINT('',(2.39275581664063,-1.28027302938979,0.9));
#11924=CARTESIAN_POINT('',(1.82679491924311,-0.3,0.6));
#11925=CARTESIAN_POINT('',(1.82679491924311,-0.3,0.9));
#11926=CARTESIAN_POINT('',(1.65358983848622,4.24230095489963E-17,0.6));
#11927=CARTESIAN_POINT('Origin',(2.17320508075689,-0.3,0.9));
#11928=CARTESIAN_POINT('',(2.17320508075689,-0.3,0.9));
#11929=CARTESIAN_POINT('',(4.52365121072543,-0.3,0.9));
#11930=CARTESIAN_POINT('',(2.17320508075689,-0.3,0.6));
#11931=CARTESIAN_POINT('',(2.17320508075689,-0.3,0.9));
#11932=CARTESIAN_POINT('',(1.82679491924311,-0.3,0.6));
#11933=CARTESIAN_POINT('Origin',(2.34641016151378,0.,0.9));
#11934=CARTESIAN_POINT('',(2.9123710589113,0.980273029389787,0.9));
#11935=CARTESIAN_POINT('',(2.17320508075689,-0.3,0.6));
#11936=CARTESIAN_POINT('Origin',(2.,5.55111512312578E-17,0.6));
#11937=CARTESIAN_POINT('',(1.83,-2.0818995585505E-17,0.6));
#11938=CARTESIAN_POINT('Origin',(2.,0.,0.6));
#11939=CARTESIAN_POINT('Origin',(2.,0.,0.45));
#11940=CARTESIAN_POINT('',(1.83,-2.0818995585505E-17,0.32));
#11941=CARTESIAN_POINT('',(1.83,2.0818995585505E-17,0.45));
#11942=CARTESIAN_POINT('Origin',(2.,0.,0.32));
#11943=CARTESIAN_POINT('Origin',(11.2,0.,0.45));
#11944=CARTESIAN_POINT('',(11.03,-2.0818995585505E-17,0.32));
#11945=CARTESIAN_POINT('',(11.03,2.0818995585505E-17,0.45));
#11946=CARTESIAN_POINT('Origin',(11.2,0.,0.32));
#11947=CARTESIAN_POINT('Origin',(12.4,-0.72,0.32));
#11948=CARTESIAN_POINT('',(0.200274469199584,-0.72,0.));
#11949=CARTESIAN_POINT('',(0.217044958570157,-0.72,0.32));
#11950=CARTESIAN_POINT('',(0.225070308370679,-0.72,0.473132796510599));
#11951=CARTESIAN_POINT('',(0.,-0.72,0.));
#11952=CARTESIAN_POINT('',(9.63649764092939,-0.72,0.));
#11953=CARTESIAN_POINT('',(0.0167704893705732,-0.72,0.32));
#11954=CARTESIAN_POINT('',(0.0253444014197637,-0.72,0.483599987759188));
#11955=CARTESIAN_POINT('',(-0.1,-0.72,0.32));
#11956=CARTESIAN_POINT('Origin',(12.4,-0.72,0.32));
#11957=CARTESIAN_POINT('',(0.9,-0.72,0.32));
#11958=CARTESIAN_POINT('',(0.9,-0.72,0.));
#11959=CARTESIAN_POINT('',(0.9,-0.72,0.16));
#11960=CARTESIAN_POINT('',(1.1,-0.72,0.32));
#11961=CARTESIAN_POINT('',(-0.1,-0.72,0.32));
#11962=CARTESIAN_POINT('',(1.1,-0.72,0.));
#11963=CARTESIAN_POINT('',(1.1,-0.72,0.16));
#11964=CARTESIAN_POINT('',(9.63649764092939,-0.72,0.));
#11965=CARTESIAN_POINT('Origin',(12.4,-0.72,0.32));
#11966=CARTESIAN_POINT('',(4.3,-0.72,0.32));
#11967=CARTESIAN_POINT('',(4.3,-0.72,0.));
#11968=CARTESIAN_POINT('',(4.3,-0.72,0.16));
#11969=CARTESIAN_POINT('',(4.5,-0.72,0.32));
#11970=CARTESIAN_POINT('',(-0.1,-0.72,0.32));
#11971=CARTESIAN_POINT('',(4.5,-0.72,0.));
#11972=CARTESIAN_POINT('',(4.5,-0.72,0.16));
#11973=CARTESIAN_POINT('',(9.63649764092939,-0.72,0.));
#11974=CARTESIAN_POINT('Origin',(12.4,-0.72,0.32));
#11975=CARTESIAN_POINT('',(8.7,-0.72,0.32));
#11976=CARTESIAN_POINT('',(8.7,-0.72,0.));
#11977=CARTESIAN_POINT('',(8.7,-0.72,0.16));
#11978=CARTESIAN_POINT('',(8.9,-0.72,0.32));
#11979=CARTESIAN_POINT('',(-0.1,-0.72,0.32));
#11980=CARTESIAN_POINT('',(8.9,-0.72,0.));
#11981=CARTESIAN_POINT('',(8.9,-0.72,0.16));
#11982=CARTESIAN_POINT('',(9.63649764092939,-0.72,0.));
#11983=CARTESIAN_POINT('Origin',(-0.0999999999999996,0.72,0.32));
#11984=CARTESIAN_POINT('',(0.217044958570158,0.72,0.32));
#11985=CARTESIAN_POINT('',(0.200274469199584,0.72,0.));
#11986=CARTESIAN_POINT('',(0.207951231396534,0.72,0.146481348799182));
#11987=CARTESIAN_POINT('',(0.0167704893705736,0.72,0.32));
#11988=CARTESIAN_POINT('',(12.4,0.72,0.32));
#11989=CARTESIAN_POINT('',(0.,0.72,0.));
#11990=CARTESIAN_POINT('',(0.00822532444561912,0.72,0.156948540047771));
#11991=CARTESIAN_POINT('',(3.38649764092939,0.72,0.));
#11992=CARTESIAN_POINT('Origin',(-0.0999999999999996,0.72,0.32));
#11993=CARTESIAN_POINT('',(0.9,0.72,0.));
#11994=CARTESIAN_POINT('',(0.9,0.72,0.32));
#11995=CARTESIAN_POINT('',(0.9,0.72,0.16));
#11996=CARTESIAN_POINT('',(1.1,0.72,0.));
#11997=CARTESIAN_POINT('',(3.38649764092939,0.72,0.));
#11998=CARTESIAN_POINT('',(1.1,0.72,0.32));
#11999=CARTESIAN_POINT('',(1.1,0.72,0.16));
#12000=CARTESIAN_POINT('',(12.4,0.72,0.32));
#12001=CARTESIAN_POINT('Origin',(-0.0999999999999996,0.72,0.32));
#12002=CARTESIAN_POINT('',(4.3,0.72,0.));
#12003=CARTESIAN_POINT('',(4.3,0.72,0.32));
#12004=CARTESIAN_POINT('',(4.3,0.72,0.16));
#12005=CARTESIAN_POINT('',(4.5,0.72,0.));
#12006=CARTESIAN_POINT('',(3.38649764092939,0.72,0.));
#12007=CARTESIAN_POINT('',(4.5,0.72,0.32));
#12008=CARTESIAN_POINT('',(4.5,0.72,0.16));
#12009=CARTESIAN_POINT('',(12.4,0.72,0.32));
#12010=CARTESIAN_POINT('Origin',(6.15,0.,0.32));
#12011=CARTESIAN_POINT('',(1.6,-4.89858719658941E-17,0.32));
#12012=CARTESIAN_POINT('Origin',(2.,0.,0.32));
#12013=CARTESIAN_POINT('Origin',(6.15,0.,0.32));
#12014=CARTESIAN_POINT('',(10.8,-4.89858719658942E-17,0.32));
#12015=CARTESIAN_POINT('Origin',(11.2,0.,0.32));
#12016=CARTESIAN_POINT('Origin',(6.15,0.,0.32));
#12017=CARTESIAN_POINT('',(0.217044958570157,-0.75,0.32));
#12018=CARTESIAN_POINT('',(0.0167704893705736,-0.75,0.32));
#12019=CARTESIAN_POINT('Origin',(6.15,0.,0.32));
#12020=CARTESIAN_POINT('',(0.9,0.696450594095222,0.32));
#12021=CARTESIAN_POINT('',(1.1,-0.696450594095222,0.32));
#12022=CARTESIAN_POINT('Origin',(6.15,0.,0.32));
#12023=CARTESIAN_POINT('',(4.3,0.742407407407408,0.32));
#12024=CARTESIAN_POINT('',(4.5,-0.742407407407408,0.32));
#12025=CARTESIAN_POINT('Origin',(6.15,0.,0.32));
#12026=CARTESIAN_POINT('',(8.7,0.72,0.32));
#12027=CARTESIAN_POINT('',(8.7,0.844259259259259,0.32));
#12028=CARTESIAN_POINT('',(8.9,0.72,0.32));
#12029=CARTESIAN_POINT('',(12.4,0.72,0.32));
#12030=CARTESIAN_POINT('',(8.9,-0.844259259259259,0.32));
#12031=CARTESIAN_POINT('Origin',(-0.0999999999999996,0.72,0.32));
#12032=CARTESIAN_POINT('',(8.7,0.72,0.));
#12033=CARTESIAN_POINT('',(8.7,0.72,0.16));
#12034=CARTESIAN_POINT('',(8.9,0.72,0.));
#12035=CARTESIAN_POINT('',(3.38649764092939,0.72,0.));
#12036=CARTESIAN_POINT('',(8.9,0.72,0.16));
#12037=CARTESIAN_POINT('Origin',(12.4,1.99376954809806,0.));
#12038=CARTESIAN_POINT('',(12.4,1.91212902562343,0.));
#12039=CARTESIAN_POINT('',(12.4,-1.91212902562343,0.));
#12040=CARTESIAN_POINT('',(12.4,1.99376954809806,0.));
#12041=CARTESIAN_POINT('',(12.4,-1.8833055216247,0.604732563714112));
#12042=CARTESIAN_POINT('Ctrl Pts',(12.4,-1.8833055216247,0.604732563714112));
#12043=CARTESIAN_POINT('Ctrl Pts',(12.4,-1.88809880980762,0.504101072758768));
#12044=CARTESIAN_POINT('Ctrl Pts',(12.4,-1.89289370245628,0.403468941627095));
#12045=CARTESIAN_POINT('Ctrl Pts',(12.4,-1.90250151416087,0.201891903194028));
#12046=CARTESIAN_POINT('Ctrl Pts',(12.4,-1.90731451170285,0.100945553925438));
#12047=CARTESIAN_POINT('Ctrl Pts',(12.4,-1.91212902562343,0.));
#12048=CARTESIAN_POINT('',(12.4,-1.78288409287054,0.7));
#12049=CARTESIAN_POINT('Ctrl Pts',(12.4000000030461,-1.78288409409899,0.7));
#12050=CARTESIAN_POINT('Ctrl Pts',(12.4000000066823,-1.79082830277209,0.699999997040196));
#12051=CARTESIAN_POINT('Ctrl Pts',(12.4000021328137,-1.79871128857748,0.699006690321208));
#12052=CARTESIAN_POINT('Ctrl Pts',(12.4000039827682,-1.8063921320806,0.697119229445379));
#12053=CARTESIAN_POINT('Ctrl Pts',(12.4000049365067,-1.81035196808589,0.69614615460905));
#12054=CARTESIAN_POINT('Ctrl Pts',(12.4000058167808,-1.81425808325963,0.694934510320783));
#12055=CARTESIAN_POINT('Ctrl Pts',(12.400006432968,-1.81808986884151,0.693492707237305));
#12056=CARTESIAN_POINT('Ctrl Pts',(12.4000076352846,-1.82556652433459,0.690679432664999));
#12057=CARTESIAN_POINT('Ctrl Pts',(12.4000076271954,-1.83268048852469,0.687023315130674));
#12058=CARTESIAN_POINT('Ctrl Pts',(12.4000063864816,-1.83928589538344,0.682605693351404));
#12059=CARTESIAN_POINT('Ctrl Pts',(12.4000055969106,-1.84348947395919,0.679794387301037));
#12060=CARTESIAN_POINT('Ctrl Pts',(12.400004329084,-1.84748689691167,0.676673627174617));
#12061=CARTESIAN_POINT('Ctrl Pts',(12.4000032503406,-1.8512341074341,0.673255429390325));
#12062=CARTESIAN_POINT('Ctrl Pts',(12.4000023796213,-1.85425870830395,0.670496394655072));
#12063=CARTESIAN_POINT('Ctrl Pts',(12.4000016297172,-1.85710218072175,0.667559826261508));
#12064=CARTESIAN_POINT('Ctrl Pts',(12.4000016274617,-1.859744520612,0.664455546516084));
#12065=CARTESIAN_POINT('Ctrl Pts',(12.4000016230979,-1.86485672743849,0.658449612092435));
#12066=CARTESIAN_POINT('Ctrl Pts',(12.4000041080363,-1.86921906069885,0.651817317967817));
#12067=CARTESIAN_POINT('Ctrl Pts',(12.40000495371,-1.8727702927896,0.64472299566344));
#12068=CARTESIAN_POINT('Ctrl Pts',(12.4000050555652,-1.8731980125259,0.643868536819953));
#12069=CARTESIAN_POINT('Ctrl Pts',(12.4000051394069,-1.87361391018412,0.643007349425002));
#12070=CARTESIAN_POINT('Ctrl Pts',(12.4000052029357,-1.87401783114888,0.642139703315781));
#12071=CARTESIAN_POINT('Ctrl Pts',(12.4000057294153,-1.87736522853405,0.634949295858174));
#12072=CARTESIAN_POINT('Ctrl Pts',(12.4000043880804,-1.87985460663586,0.627401584261416));
#12073=CARTESIAN_POINT('Ctrl Pts',(12.4000025112034,-1.88143175301701,0.619663949188762));
#12074=CARTESIAN_POINT('Ctrl Pts',(12.4000013193515,-1.88243327046239,0.614750406220363));
#12075=CARTESIAN_POINT('Ctrl Pts',(12.4,-1.88306607129604,0.609759643802656));
#12076=CARTESIAN_POINT('Ctrl Pts',(12.4,-1.8833055216247,0.604732563714112));
#12077=CARTESIAN_POINT('',(12.4,1.78288409287164,0.7));
#12078=CARTESIAN_POINT('',(12.4,0.99688477404903,0.7));
#12079=CARTESIAN_POINT('',(12.4,1.8833055216247,0.604732563714112));
#12080=CARTESIAN_POINT('Ctrl Pts',(12.4,1.8833055216247,0.604732563714112));
#12081=CARTESIAN_POINT('Ctrl Pts',(12.4,1.88292893537322,0.612638709665068));
#12082=CARTESIAN_POINT('Ctrl Pts',(12.4000029905988,1.88158186833012,0.620459457162159));
#12083=CARTESIAN_POINT('Ctrl Pts',(12.400004351969,1.87934739482834,0.62803467841275));
#12084=CARTESIAN_POINT('Ctrl Pts',(12.4000050124983,1.87826324073514,0.631710133556493));
#12085=CARTESIAN_POINT('Ctrl Pts',(12.4000053733669,1.87696936339782,0.63532777623417));
#12086=CARTESIAN_POINT('Ctrl Pts',(12.4000053391329,1.87547104796815,0.638868146717817));
#12087=CARTESIAN_POINT('Ctrl Pts',(12.4000052683671,1.872373843052,0.646186534188034));
#12088=CARTESIAN_POINT('Ctrl Pts',(12.4000032465668,1.86844110215533,0.653093304890266));
#12089=CARTESIAN_POINT('Ctrl Pts',(12.4000021327941,1.86374151467895,0.659427433016556));
#12090=CARTESIAN_POINT('Ctrl Pts',(12.4000018304335,1.86246569800928,0.66114698527342));
#12091=CARTESIAN_POINT('Ctrl Pts',(12.4000016226794,1.86113309763036,0.662824214875179));
#12092=CARTESIAN_POINT('Ctrl Pts',(12.400001625255,1.85974452038344,0.664455546516227));
#12093=CARTESIAN_POINT('Ctrl Pts',(12.4000016287814,1.85784336180007,0.666689070188443));
#12094=CARTESIAN_POINT('Ctrl Pts',(12.400002024929,1.85583728779192,0.668836587948716));
#12095=CARTESIAN_POINT('Ctrl Pts',(12.4000025639666,1.85373364862045,0.670894373083513));
#12096=CARTESIAN_POINT('Ctrl Pts',(12.400004021536,1.84804536272624,0.676458668669153));
#12097=CARTESIAN_POINT('Ctrl Pts',(12.4000062945443,1.84171268252251,0.681305055194542));
#12098=CARTESIAN_POINT('Ctrl Pts',(12.4000070319583,1.83490078417639,0.685381489016216));
#12099=CARTESIAN_POINT('Ctrl Pts',(12.4000075068619,1.8305138392177,0.688006761722114));
#12100=CARTESIAN_POINT('Ctrl Pts',(12.4000074483741,1.82592714021755,0.69031203082117));
#12101=CARTESIAN_POINT('Ctrl Pts',(12.4000068708525,1.82117863971551,0.692273867243687));
#12102=CARTESIAN_POINT('Ctrl Pts',(12.4000059767178,1.81382688138917,0.695311236040001));
#12103=CARTESIAN_POINT('Ctrl Pts',(12.4000038254996,1.80617119073902,0.697493343451155));
#12104=CARTESIAN_POINT('Ctrl Pts',(12.4000020685374,1.7983596509798,0.698751345219246));
#12105=CARTESIAN_POINT('Ctrl Pts',(12.4000009204513,1.79325520389048,0.699573385900268));
#12106=CARTESIAN_POINT('Ctrl Pts',(12.400000005426,1.78808359082883,0.699999998062804));
#12107=CARTESIAN_POINT('Ctrl Pts',(12.4000000030461,1.78288409409899,0.7));
#12108=CARTESIAN_POINT('Ctrl Pts',(12.4,1.91212902562343,0.));
#12109=CARTESIAN_POINT('Ctrl Pts',(12.4,1.90731404243129,0.1009553931071));
#12110=CARTESIAN_POINT('Ctrl Pts',(12.4,1.9025005759122,0.201911581737034));
#12111=CARTESIAN_POINT('Ctrl Pts',(12.4,1.89289276481806,0.403488620176902));
#12112=CARTESIAN_POINT('Ctrl Pts',(12.4,1.88809834114759,0.504110911924693));
#12113=CARTESIAN_POINT('Ctrl Pts',(12.4,1.8833055216247,0.604732563714112));
#12114=CARTESIAN_POINT('Origin',(8.9,-1.68851851851852,0.));
#12115=CARTESIAN_POINT('',(8.9,1.62420669932031,0.));
#12116=CARTESIAN_POINT('',(8.9,-1.68851851851852,0.));
#12117=CARTESIAN_POINT('',(8.9,1.59320117118329,0.605106081470792));
#12118=CARTESIAN_POINT('Ctrl Pts',(8.9,1.59320117118329,0.605106081470792));
#12119=CARTESIAN_POINT('Ctrl Pts',(8.9,1.59837103562161,0.504197738990529));
#12120=CARTESIAN_POINT('Ctrl Pts',(8.9,1.60354126123154,0.403288838380538));
#12121=CARTESIAN_POINT('Ctrl Pts',(8.9,1.61387642009944,0.201587196710533));
#12122=CARTESIAN_POINT('Ctrl Pts',(8.9,1.61904141157348,0.100793304842659));
#12123=CARTESIAN_POINT('Ctrl Pts',(8.9,1.62420669932031,0.));
#12124=CARTESIAN_POINT('',(8.9,1.49312521822106,0.7));
#12125=CARTESIAN_POINT('Ctrl Pts',(8.9,1.49312521822106,0.7));
#12126=CARTESIAN_POINT('Ctrl Pts',(8.9,1.50104136823484,0.7));
#12127=CARTESIAN_POINT('Ctrl Pts',(8.90000131173634,1.50889623314995,0.699007530025307));
#12128=CARTESIAN_POINT('Ctrl Pts',(8.90000245364087,1.51654949575132,0.697121675771258));
#12129=CARTESIAN_POINT('Ctrl Pts',(8.9000030153269,1.52031402289636,0.696194051841344));
#12130=CARTESIAN_POINT('Ctrl Pts',(8.90000353645954,1.52402976767023,0.695049421358208));
#12131=CARTESIAN_POINT('Ctrl Pts',(8.90000391188735,1.52767894577544,0.693695149285802));
#12132=CARTESIAN_POINT('Ctrl Pts',(8.90000468147812,1.53515940869299,0.690919022244083));
#12133=CARTESIAN_POINT('Ctrl Pts',(8.90000470661952,1.54227958804117,0.687295426711095));
#12134=CARTESIAN_POINT('Ctrl Pts',(8.9000039635008,1.54889410374269,0.682907715777054));
#12135=CARTESIAN_POINT('Ctrl Pts',(8.90000349228854,1.55308837416723,0.680125464281631));
#12136=CARTESIAN_POINT('Ctrl Pts',(8.90000272405863,1.55707914411963,0.677034908766328));
#12137=CARTESIAN_POINT('Ctrl Pts',(8.90000205379677,1.56082314136721,0.673648333128258));
#12138=CARTESIAN_POINT('Ctrl Pts',(8.90000149471997,1.56394607304962,0.670823532879853));
#12139=CARTESIAN_POINT('Ctrl Pts',(8.90000100172653,1.56687805273397,0.667809941545923));
#12140=CARTESIAN_POINT('Ctrl Pts',(8.90000100003,1.56959740049228,0.664618488856983));
#12141=CARTESIAN_POINT('Ctrl Pts',(8.90000099684156,1.57470809805256,0.658620525035968));
#12142=CARTESIAN_POINT('Ctrl Pts',(8.90000253934467,1.57907071782202,0.651995745956818));
#12143=CARTESIAN_POINT('Ctrl Pts',(8.90000305932469,1.58262507990443,0.644909256877938));
#12144=CARTESIAN_POINT('Ctrl Pts',(8.90000311559331,1.58300970826793,0.644142406277414));
#12145=CARTESIAN_POINT('Ctrl Pts',(8.9000031627798,1.58338482682255,0.643370127200485));
#12146=CARTESIAN_POINT('Ctrl Pts',(8.90000319981124,1.58375032531468,0.642592615892991));
#12147=CARTESIAN_POINT('Ctrl Pts',(8.90000354178946,1.58712563340961,0.635412448897651));
#12148=CARTESIAN_POINT('Ctrl Pts',(8.90000272882427,1.58964525157545,0.627871187463612));
#12149=CARTESIAN_POINT('Ctrl Pts',(8.90000156924769,1.59125549206429,0.620136848214628));
#12150=CARTESIAN_POINT('Ctrl Pts',(8.90000082792478,1.59228492658837,0.615192247765769));
#12151=CARTESIAN_POINT('Ctrl Pts',(8.89999999997262,1.59294182914154,0.610168076493048));
#12152=CARTESIAN_POINT('Ctrl Pts',(8.9000000009702,1.5932011715731,0.605106081469384));
#12153=CARTESIAN_POINT('',(8.9,-1.49312521822001,0.7));
#12154=CARTESIAN_POINT('',(8.9,-0.844259259259259,0.7));
#12155=CARTESIAN_POINT('',(8.9,-1.59320117118329,0.605106081470792));
#12156=CARTESIAN_POINT('Ctrl Pts',(8.90000000097019,-1.5932011715731,0.605106081469384));
#12157=CARTESIAN_POINT('Ctrl Pts',(8.89999999941083,-1.59279578158415,0.613018716877257));
#12158=CARTESIAN_POINT('Ctrl Pts',(8.90000185372291,-1.59142151714118,0.620841302874248));
#12159=CARTESIAN_POINT('Ctrl Pts',(8.90000269095591,-1.58916270068609,0.628413601005994));
#12160=CARTESIAN_POINT('Ctrl Pts',(8.90000316003867,-1.58789713677684,0.632656188846207));
#12161=CARTESIAN_POINT('Ctrl Pts',(8.90000337414869,-1.58635289833986,0.636820251299613));
#12162=CARTESIAN_POINT('Ctrl Pts',(8.90000326408749,-1.58453800492682,0.640875626603871));
#12163=CARTESIAN_POINT('Ctrl Pts',(8.9000030675631,-1.58129734600662,0.648116871770122));
#12164=CARTESIAN_POINT('Ctrl Pts',(8.90000169351568,-1.5772322800227,0.654932667693845));
#12165=CARTESIAN_POINT('Ctrl Pts',(8.90000116172667,-1.57240747726376,0.66116027211862));
#12166=CARTESIAN_POINT('Ctrl Pts',(8.90000106146602,-1.57149783490479,0.662334391157823));
#12167=CARTESIAN_POINT('Ctrl Pts',(8.90000099955281,-1.57056105641498,0.663487533005214));
#12168=CARTESIAN_POINT('Ctrl Pts',(8.90000100072893,-1.56959740053727,0.664618488856962));
#12169=CARTESIAN_POINT('Ctrl Pts',(8.9000010030487,-1.56769671285427,0.666849154291726));
#12170=CARTESIAN_POINT('Ctrl Pts',(8.90000124864079,-1.56569149899762,0.668993559652069));
#12171=CARTESIAN_POINT('Ctrl Pts',(8.90000158179872,-1.56358911460694,0.671047966011734));
#12172=CARTESIAN_POINT('Ctrl Pts',(8.90000248280001,-1.55790336961918,0.676603957919834));
#12173=CARTESIAN_POINT('Ctrl Pts',(8.90000387848177,-1.55157399841983,0.681441805123218));
#12174=CARTESIAN_POINT('Ctrl Pts',(8.90000432886686,-1.54476515293017,0.68550782533293));
#12175=CARTESIAN_POINT('Ctrl Pts',(8.9000046162921,-1.54041990676133,0.688102664467623));
#12176=CARTESIAN_POINT('Ctrl Pts',(8.90000458123012,-1.53587841548674,0.69038248607508));
#12177=CARTESIAN_POINT('Ctrl Pts',(8.90000422571091,-1.53117752164703,0.692323975790708));
#12178=CARTESIAN_POINT('Ctrl Pts',(8.90000367147839,-1.52384911813356,0.695350638493274));
#12179=CARTESIAN_POINT('Ctrl Pts',(8.9000023358238,-1.51621796414731,0.697522741667433));
#12180=CARTESIAN_POINT('Ctrl Pts',(8.90000125519218,-1.50843132129101,0.698770821080692));
#12181=CARTESIAN_POINT('Ctrl Pts',(8.90000055451733,-1.5033825102871,0.699580068042664));
#12182=CARTESIAN_POINT('Ctrl Pts',(8.9,-1.49826772866746,0.7));
#12183=CARTESIAN_POINT('Ctrl Pts',(8.9,-1.49312521822106,0.7));
#12184=CARTESIAN_POINT('',(8.9,-1.62420669932031,0.));
#12185=CARTESIAN_POINT('Ctrl Pts',(8.9,-1.62420669932031,0.));
#12186=CARTESIAN_POINT('Ctrl Pts',(8.9,-1.61904139377919,0.100793652073202));
#12187=CARTESIAN_POINT('Ctrl Pts',(8.9,-1.61387638451174,0.201587891198165));
#12188=CARTESIAN_POINT('Ctrl Pts',(8.9,-1.60354122564866,0.403289532862703));
#12189=CARTESIAN_POINT('Ctrl Pts',(8.9,-1.59837101783099,0.50419808623799));
#12190=CARTESIAN_POINT('Ctrl Pts',(8.9,-1.59320117118329,0.605106081470792));
#12191=CARTESIAN_POINT('',(8.9,-1.68851851851852,0.));
#12192=CARTESIAN_POINT('Origin',(4.5,-1.48481481481482,0.));
#12193=CARTESIAN_POINT('',(4.5,1.41772989878425,0.));
#12194=CARTESIAN_POINT('',(4.5,-1.48481481481482,0.));
#12195=CARTESIAN_POINT('',(4.5,1.38566996325095,0.605286533624017));
#12196=CARTESIAN_POINT('Ctrl Pts',(4.5,1.38566996325095,0.605286533624017));
#12197=CARTESIAN_POINT('Ctrl Pts',(4.5,1.3910232158183,0.504222354021684));
#12198=CARTESIAN_POINT('Ctrl Pts',(4.5,1.39637635187357,0.403158168247774));
#12199=CARTESIAN_POINT('Ctrl Pts',(4.5,1.4070629957395,0.201395990303158));
#12200=CARTESIAN_POINT('Ctrl Pts',(4.5,1.41239650438775,0.100697998177668));
#12201=CARTESIAN_POINT('Ctrl Pts',(4.5,1.41772989878425,0.));
#12202=CARTESIAN_POINT('',(4.5,1.28575421950843,0.7));
#12203=CARTESIAN_POINT('Ctrl Pts',(4.5,1.28575421950843,0.7));
#12204=CARTESIAN_POINT('Ctrl Pts',(4.5,1.29366545802379,0.7));
#12205=CARTESIAN_POINT('Ctrl Pts',(4.50000067540813,1.30151306508378,0.699006020085879));
#12206=CARTESIAN_POINT('Ctrl Pts',(4.50000126278178,1.30915682219698,0.697118891599074));
#12207=CARTESIAN_POINT('Ctrl Pts',(4.50000159346398,1.31346013814185,0.696056467716811));
#12208=CARTESIAN_POINT('Ctrl Pts',(4.50000189442328,1.31769890045703,0.694709922559592));
#12209=CARTESIAN_POINT('Ctrl Pts',(4.50000208642664,1.32184639782974,0.693090275295953));
#12210=CARTESIAN_POINT('Ctrl Pts',(4.50000243009859,1.32927011415192,0.690191225399894));
#12211=CARTESIAN_POINT('Ctrl Pts',(4.50000235826664,1.33632110693134,0.686451804482762));
#12212=CARTESIAN_POINT('Ctrl Pts',(4.50000192249634,1.34285330390028,0.681953677325188));
#12213=CARTESIAN_POINT('Ctrl Pts',(4.5000016824508,1.3464515866709,0.679475868782656));
#12214=CARTESIAN_POINT('Ctrl Pts',(4.50000134086274,1.34989218134371,0.676766953538005));
#12215=CARTESIAN_POINT('Ctrl Pts',(4.50000103767597,1.35314674504257,0.67383503027087));
#12216=CARTESIAN_POINT('Ctrl Pts',(4.50000074242034,1.35631617169348,0.670979804009792));
#12217=CARTESIAN_POINT('Ctrl Pts',(4.50000047986374,1.35928994516467,0.667930335702103));
#12218=CARTESIAN_POINT('Ctrl Pts',(4.5000004798165,1.36204555935344,0.66469809744354));
#12219=CARTESIAN_POINT('Ctrl Pts',(4.5000004797289,1.36715559606013,0.658704204607119));
#12220=CARTESIAN_POINT('Ctrl Pts',(4.50000128456446,1.3715183542993,0.652083197653858));
#12221=CARTESIAN_POINT('Ctrl Pts',(4.50000155892095,1.37507421485048,0.645000595057188));
#12222=CARTESIAN_POINT('Ctrl Pts',(4.50000158702893,1.37543851484667,0.644274978272754));
#12223=CARTESIAN_POINT('Ctrl Pts',(4.50000161091379,1.37579430519483,0.643544496675346));
#12224=CARTESIAN_POINT('Ctrl Pts',(4.50000163009343,1.37614149316233,0.642809317076966));
#12225=CARTESIAN_POINT('Ctrl Pts',(4.50000181728783,1.37953006709248,0.635633923185928));
#12226=CARTESIAN_POINT('Ctrl Pts',(4.50000140772507,1.38206400387968,0.628095594687559));
#12227=CARTESIAN_POINT('Ctrl Pts',(4.50000081194859,1.38368993781387,0.620362729373495));
#12228=CARTESIAN_POINT('Ctrl Pts',(4.50000042990035,1.38473258588096,0.615403944208116));
#12229=CARTESIAN_POINT('Ctrl Pts',(4.49999999988018,1.38540098970406,0.610364492806037));
#12230=CARTESIAN_POINT('Ctrl Pts',(4.50000000014037,1.38566996330298,0.605286533623957));
#12231=CARTESIAN_POINT('',(4.5,-1.28575421950842,0.7));
#12232=CARTESIAN_POINT('',(4.5,-0.742407407407408,0.7));
#12233=CARTESIAN_POINT('',(4.5,-1.38566996325095,0.605286533624017));
#12234=CARTESIAN_POINT('Ctrl Pts',(4.50000000014037,-1.38566996330298,0.605286533623957));
#12235=CARTESIAN_POINT('Ctrl Pts',(4.49999999973491,-1.38525081272033,0.613199687771457));
#12236=CARTESIAN_POINT('Ctrl Pts',(4.50000095642016,-1.38386419754969,0.62102180968747));
#12237=CARTESIAN_POINT('Ctrl Pts',(4.50000138305812,-1.38159414679432,0.628592503408469));
#12238=CARTESIAN_POINT('Ctrl Pts',(4.50000162118259,-1.38032713666619,0.632818023740444));
#12239=CARTESIAN_POINT('Ctrl Pts',(4.50000172745986,-1.37878391728058,0.636965253716347));
#12240=CARTESIAN_POINT('Ctrl Pts',(4.50000166716583,-1.37697237493585,0.641004309729874));
#12241=CARTESIAN_POINT('Ctrl Pts',(4.50000155916287,-1.37372741146613,0.648239354085419));
#12242=CARTESIAN_POINT('Ctrl Pts',(4.50000084040372,-1.36965973349804,0.655049237033139));
#12243=CARTESIAN_POINT('Ctrl Pts',(4.50000056390271,-1.36483316768901,0.661270759279915));
#12244=CARTESIAN_POINT('Ctrl Pts',(4.50000051219424,-1.36393055121024,0.662434246679675));
#12245=CARTESIAN_POINT('Ctrl Pts',(4.50000048023544,-1.3630012658104,0.663577087492372));
#12246=CARTESIAN_POINT('Ctrl Pts',(4.50000048056391,-1.36204555937839,0.664698097443534));
#12247=CARTESIAN_POINT('Ctrl Pts',(4.50000048121673,-1.36014610273268,0.666926093123284));
#12248=CARTESIAN_POINT('Ctrl Pts',(4.50000060829837,-1.35814231322364,0.669067903674665));
#12249=CARTESIAN_POINT('Ctrl Pts',(4.50000078085101,-1.35604151212276,0.671119765431539));
#12250=CARTESIAN_POINT('Ctrl Pts',(4.50000124774248,-1.3503571825734,0.676671675324794));
#12251=CARTESIAN_POINT('Ctrl Pts',(4.50000197143062,-1.34402953514766,0.681505303070731));
#12252=CARTESIAN_POINT('Ctrl Pts',(4.50000220836427,-1.33722229030693,0.685566265232058));
#12253=CARTESIAN_POINT('Ctrl Pts',(4.50000235894787,-1.33289593407788,0.688147216755564));
#12254=CARTESIAN_POINT('Ctrl Pts',(4.50000234488938,-1.32837489877041,0.690415387400166));
#12255=CARTESIAN_POINT('Ctrl Pts',(4.50000216490635,-1.32369554581057,0.69234752884452));
#12256=CARTESIAN_POINT('Ctrl Pts',(4.50000188343739,-1.31637767466938,0.695369135087455));
#12257=CARTESIAN_POINT('Ctrl Pts',(4.50000119588393,-1.3087575932273,0.697536490026807));
#12258=CARTESIAN_POINT('Ctrl Pts',(4.50000064127173,-1.30098224657147,0.698779892333419));
#12259=CARTESIAN_POINT('Ctrl Pts',(4.50000028296845,-1.29595903898196,0.699583183579437));
#12260=CARTESIAN_POINT('Ctrl Pts',(4.5,-1.29087043558603,0.7));
#12261=CARTESIAN_POINT('Ctrl Pts',(4.5,-1.28575421950843,0.7));
#12262=CARTESIAN_POINT('',(4.5,-1.41772989878425,0.));
#12263=CARTESIAN_POINT('Ctrl Pts',(4.5,-1.41772989878425,0.));
#12264=CARTESIAN_POINT('Ctrl Pts',(4.5,-1.41239649634988,0.100698149937961));
#12265=CARTESIAN_POINT('Ctrl Pts',(4.5,-1.40706297966336,0.201396293824709));
#12266=CARTESIAN_POINT('Ctrl Pts',(4.5,-1.39637633579674,0.403158471769294));
#12267=CARTESIAN_POINT('Ctrl Pts',(4.5,-1.39102320777973,0.504222505781934));
#12268=CARTESIAN_POINT('Ctrl Pts',(4.5,-1.38566996325095,0.605286533624017));
#12269=CARTESIAN_POINT('',(4.5,-1.48481481481482,0.));
#12270=CARTESIAN_POINT('Origin',(1.1,-1.39290118819044,0.));
#12271=CARTESIAN_POINT('',(1.1,1.324891758307,0.));
#12272=CARTESIAN_POINT('',(1.1,-1.39290118819044,0.));
#12273=CARTESIAN_POINT('',(1.10000000295569,1.29254692766489,0.605334652628491));
#12274=CARTESIAN_POINT('Ctrl Pts',(1.10000000295569,1.29254692766489,0.605334652628491));
#12275=CARTESIAN_POINT('Ctrl Pts',(1.10000000295569,1.29794978210809,0.504228164786351));
#12276=CARTESIAN_POINT('Ctrl Pts',(1.1,1.30335245345465,0.403121008362245));
#12277=CARTESIAN_POINT('Ctrl Pts',(1.1,1.31413403739463,0.20134322693425));
#12278=CARTESIAN_POINT('Ctrl Pts',(1.1,1.31951302132877,0.100671299071668));
#12279=CARTESIAN_POINT('Ctrl Pts',(1.1,1.324891758307,0.));
#12280=CARTESIAN_POINT('Ctrl Pts',(1.1,1.19266190204553,0.7));
#12281=CARTESIAN_POINT('Ctrl Pts',(1.1,1.20057109129252,0.7));
#12282=CARTESIAN_POINT('Ctrl Pts',(1.10000046829629,1.20841685974333,0.699006220526237));
#12283=CARTESIAN_POINT('Ctrl Pts',(1.10000087277688,1.21605887983377,0.697119382842322));
#12284=CARTESIAN_POINT('Ctrl Pts',(1.10000109992184,1.22035042410288,0.696059787689036));
#12285=CARTESIAN_POINT('Ctrl Pts',(1.10000130563842,1.22457776983048,0.694717521940989));
#12286=CARTESIAN_POINT('Ctrl Pts',(1.10000143498593,1.22871439246446,0.693103507978966));
#12287=CARTESIAN_POINT('Ctrl Pts',(1.10000166711622,1.23613807995602,0.690206957744321));
#12288=CARTESIAN_POINT('Ctrl Pts',(1.10000160692769,1.24318920265812,0.686469797174223));
#12289=CARTESIAN_POINT('Ctrl Pts',(1.10000129432656,1.24972159507123,0.681973692132557));
#12290=CARTESIAN_POINT('Ctrl Pts',(1.10000112259081,1.25331033895651,0.679503636989594));
#12291=CARTESIAN_POINT('Ctrl Pts',(1.10000088087184,1.25674225826706,0.676803638555143));
#12292=CARTESIAN_POINT('Ctrl Pts',(1.10000066684112,1.25998923415267,0.673881729486736));
#12293=CARTESIAN_POINT('Ctrl Pts',(1.100000457217,1.26316935916797,0.671019978599686));
#12294=CARTESIAN_POINT('Ctrl Pts',(1.1000002715704,1.26615273734033,0.667962699881477));
#12295=CARTESIAN_POINT('Ctrl Pts',(1.1000002731257,1.2689166530284,0.664721467295484));
#12296=CARTESIAN_POINT('Ctrl Pts',(1.10000027600127,1.2740268283512,0.658728785663437));
#12297=CARTESIAN_POINT('Ctrl Pts',(1.10000085014601,1.27838972527875,0.652108677049879));
#12298=CARTESIAN_POINT('Ctrl Pts',(1.1000010530947,1.28194599975408,0.64502688444408));
#12299=CARTESIAN_POINT('Ctrl Pts',(1.10000107362034,1.2823056710724,0.644310652415237));
#12300=CARTESIAN_POINT('Ctrl Pts',(1.10000109127028,1.28265705236355,0.643589678557342));
#12301=CARTESIAN_POINT('Ctrl Pts',(1.10000110571348,1.28300005475086,0.642864123553892));
#12302=CARTESIAN_POINT('Ctrl Pts',(1.10000124853573,1.28639184812822,0.635689442715943));
#12303=CARTESIAN_POINT('Ctrl Pts',(1.10000097361067,1.28892914698194,0.628151301589031));
#12304=CARTESIAN_POINT('Ctrl Pts',(1.10000056283738,1.29055881622654,0.620418355899457));
#12305=CARTESIAN_POINT('Ctrl Pts',(1.10000029930222,1.29160434466024,0.615457217544876));
#12306=CARTESIAN_POINT('Ctrl Pts',(1.0999999999818,1.29227543558766,0.610415225971447));
#12307=CARTESIAN_POINT('Ctrl Pts',(1.1000000000255,1.29254692753179,0.605334652628598));
#12308=CARTESIAN_POINT('',(1.10000000295569,-1.29254692766489,0.605334652628491));
#12309=CARTESIAN_POINT('Ctrl Pts',(1.1000000000255,-1.29254692753179,0.605334652628598));
#12310=CARTESIAN_POINT('Ctrl Pts',(1.09999999995744,-1.29212405100831,0.613248166229861));
#12311=CARTESIAN_POINT('Ctrl Pts',(1.10000066442022,-1.29073420569755,0.621070584654331));
#12312=CARTESIAN_POINT('Ctrl Pts',(1.10000095378343,-1.28846118610397,0.628641296001913));
#12313=CARTESIAN_POINT('Ctrl Pts',(1.10000111506646,-1.28719426797524,0.632861000698125));
#12314=CARTESIAN_POINT('Ctrl Pts',(1.10000118318417,-1.28565198202118,0.637002542581089));
#12315=CARTESIAN_POINT('Ctrl Pts',(1.10000113489265,-1.28384214455607,0.641036116698538));
#12316=CARTESIAN_POINT('Ctrl Pts',(1.10000104828677,-1.28059638744501,0.648269916488365));
#12317=CARTESIAN_POINT('Ctrl Pts',(1.10000053334783,-1.27652829029495,0.655078571385522));
#12318=CARTESIAN_POINT('Ctrl Pts',(1.10000033433257,-1.27170133822839,0.661298646557671));
#12319=CARTESIAN_POINT('Ctrl Pts',(1.10000029715544,-1.27079963749419,0.662460590217389));
#12320=CARTESIAN_POINT('Ctrl Pts',(1.10000027400485,-1.26987132743055,0.663601924550879));
#12321=CARTESIAN_POINT('Ctrl Pts',(1.10000027368829,-1.26891665304159,0.664721467295481));
#12322=CARTESIAN_POINT('Ctrl Pts',(1.10000027305905,-1.2670190620795,0.666946764442229));
#12323=CARTESIAN_POINT('Ctrl Pts',(1.10000036187052,-1.26501734165944,0.669086014589825));
#12324=CARTESIAN_POINT('Ctrl Pts',(1.10000048327469,-1.26291879257262,0.671135465892351));
#12325=CARTESIAN_POINT('Ctrl Pts',(1.10000081209565,-1.25723491092676,0.676686367091516));
#12326=CARTESIAN_POINT('Ctrl Pts',(1.10000132622062,-1.25090760500066,0.68151881845922));
#12327=CARTESIAN_POINT('Ctrl Pts',(1.10000150097561,-1.24410063152763,0.68557843671136));
#12328=CARTESIAN_POINT('Ctrl Pts',(1.10000161196703,-1.2397773464179,0.688156805381407));
#12329=CARTESIAN_POINT('Ctrl Pts',(1.1000016084534,-1.23525961544019,0.690422742497405));
#12330=CARTESIAN_POINT('Ctrl Pts',(1.10000148831111,-1.23058375131837,0.692353039195786));
#12331=CARTESIAN_POINT('Ctrl Pts',(1.10000130031927,-1.22326722442338,0.695373457954986));
#12332=CARTESIAN_POINT('Ctrl Pts',(1.1000008264887,-1.21564857658641,0.697539632783775));
#12333=CARTESIAN_POINT('Ctrl Pts',(1.10000044322439,-1.20787483729518,0.698781928831272));
#12334=CARTESIAN_POINT('Ctrl Pts',(1.1000001958084,-1.20285650563037,0.6995838921283));
#12335=CARTESIAN_POINT('Ctrl Pts',(1.1,-1.19777295102175,0.7));
#12336=CARTESIAN_POINT('Ctrl Pts',(1.1,-1.19266190204553,0.7));
#12337=CARTESIAN_POINT('',(1.1,-1.324891758307,0.));
#12338=CARTESIAN_POINT('Ctrl Pts',(1.1,-1.324891758307,0.));
#12339=CARTESIAN_POINT('Ctrl Pts',(1.1,-1.3195129727271,0.10067220872632));
#12340=CARTESIAN_POINT('Ctrl Pts',(1.1,-1.31413394019217,0.201345046154956));
#12341=CARTESIAN_POINT('Ctrl Pts',(1.1,-1.30335235623932,0.40312282767794));
#12342=CARTESIAN_POINT('Ctrl Pts',(1.10000000295569,-1.29794973349953,0.504229074424201));
#12343=CARTESIAN_POINT('Ctrl Pts',(1.10000000295569,-1.29254692766489,0.605334652628491));
#12344=CARTESIAN_POINT('',(1.1,-1.39290118819044,0.));
#12345=CARTESIAN_POINT('Origin',(0.199725906950915,-1.5,-0.0104671912485888));
#12346=CARTESIAN_POINT('',(0.200274469199584,1.20659878095028,0.));
#12347=CARTESIAN_POINT('',(0.200274469199585,-0.75,0.));
#12348=CARTESIAN_POINT('',(0.231993417893744,1.17491202960101,0.605233595624295));
#12349=CARTESIAN_POINT('Ctrl Pts',(0.200274469199584,1.20659878095028,-9.43255890062389E-18));
#12350=CARTESIAN_POINT('Ctrl Pts',(0.210847451958254,1.19603647956141,0.20174452921517));
#12351=CARTESIAN_POINT('Ctrl Pts',(0.221420434855641,1.18547422886796,0.403489061077219));
#12352=CARTESIAN_POINT('Ctrl Pts',(0.231993417893744,1.17491202960101,0.605233595624295));
#12353=CARTESIAN_POINT('',(0.231993417893744,-1.17491202960101,0.605233595624295));
#12354=CARTESIAN_POINT('',(0.231993417893744,-0.75,0.605233595624295));
#12355=CARTESIAN_POINT('',(0.200274469199584,-1.20659878095028,1.38777878078145E-17));
#12356=CARTESIAN_POINT('Ctrl Pts',(0.231993417893744,-1.17491202960101,
0.605233595624295));
#12357=CARTESIAN_POINT('Ctrl Pts',(0.221420434855641,-1.18547422886796,
0.40348906107722));
#12358=CARTESIAN_POINT('Ctrl Pts',(0.210847451958254,-1.19603647956141,
0.20174452921517));
#12359=CARTESIAN_POINT('Ctrl Pts',(0.200274469199584,-1.20659878095028,
2.0491421059976E-17));
#12360=CARTESIAN_POINT('',(0.200274469199585,-0.75,0.));
#12361=CARTESIAN_POINT('Origin',(6.87299528185878,-3.57834294608796E-18,
0.));
#12362=CARTESIAN_POINT('Ctrl Pts',(8.90000000000001,-1.62420669932031,-3.75133951679985E-17));
#12363=CARTESIAN_POINT('Ctrl Pts',(10.0682843079684,-1.69891080436391,-1.31961514553165E-7));
#12364=CARTESIAN_POINT('Ctrl Pts',(11.2345361392062,-1.79243531443695,-6.44452192334729E-8));
#12365=CARTESIAN_POINT('Ctrl Pts',(12.4000000002382,-1.91212902541327,2.95121624705651E-11));
#12366=CARTESIAN_POINT('Ctrl Pts',(12.4000000002382,1.91212902541327,2.95118849063386E-11));
#12367=CARTESIAN_POINT('Ctrl Pts',(11.2345361911441,1.79243531977099,-6.4445136166539E-8));
#12368=CARTESIAN_POINT('Ctrl Pts',(10.0682843567552,1.69891080748336,-1.31958638870612E-7));
#12369=CARTESIAN_POINT('Ctrl Pts',(8.9,1.62420669932031,6.39679281766448E-17));
#12370=CARTESIAN_POINT('',(8.7,1.61160179736194,0.));
#12371=CARTESIAN_POINT('',(8.7,1.68851851851852,0.));
#12372=CARTESIAN_POINT('Ctrl Pts',(8.70000000002062,1.61160179731554,-3.21507306454832E-13));
#12373=CARTESIAN_POINT('Ctrl Pts',(7.99734938728961,1.56795839277283,5.29471456843263E-9));
#12374=CARTESIAN_POINT('Ctrl Pts',(7.29393815910572,1.53097060499506,-6.44604909847991E-9));
#12375=CARTESIAN_POINT('Ctrl Pts',(6.58949465297818,1.49904250536939,-7.60372244394637E-9));
#12376=CARTESIAN_POINT('Ctrl Pts',(5.94302350041144,1.46974193664425,-8.66612477447903E-9));
#12377=CARTESIAN_POINT('Ctrl Pts',(5.29757001768168,1.44478244743454,1.79883147367388E-8));
#12378=CARTESIAN_POINT('Ctrl Pts',(4.65216233480351,1.42284617839366,3.84107779578714E-9));
#12379=CARTESIAN_POINT('Ctrl Pts',(4.60144142975536,1.4211222642714,2.72928337404163E-9));
#12380=CARTESIAN_POINT('Ctrl Pts',(4.55072080855761,1.41941704699729,1.44770501019496E-9));
#12381=CARTESIAN_POINT('Ctrl Pts',(4.50000000001737,1.41772989873549,-1.00876616052154E-12));
#12382=CARTESIAN_POINT('',(4.3,1.41116952203211,0.));
#12383=CARTESIAN_POINT('',(4.3,1.48481481481482,0.));
#12384=CARTESIAN_POINT('Ctrl Pts',(4.3,1.41116952203211,-1.0790522121662E-15));
#12385=CARTESIAN_POINT('Ctrl Pts',(3.23514221724601,1.37672428690534,3.20725535317031E-8));
#12386=CARTESIAN_POINT('Ctrl Pts',(2.16992716239601,1.34987955958158,4.63097810372671E-9));
#12387=CARTESIAN_POINT('Ctrl Pts',(1.10000000020726,1.32489175811528,-9.82792569252214E-12));
#12388=CARTESIAN_POINT('',(0.9,1.32024227787037,0.));
#12389=CARTESIAN_POINT('',(0.9,1.39290118819044,0.));
#12390=CARTESIAN_POINT('',(0.297857995688647,1.306435779838,0.));
#12391=CARTESIAN_POINT('Ctrl Pts',(0.9,1.32024227787037,-6.93889390390723E-18));
#12392=CARTESIAN_POINT('Ctrl Pts',(0.699470323836888,1.31560060380002,-4.72996299588896E-10));
#12393=CARTESIAN_POINT('Ctrl Pts',(0.498765843889866,1.3110112408976,-1.02277582142263E-13));
#12394=CARTESIAN_POINT('Ctrl Pts',(0.297857995688647,1.306435779838,-1.00157829096748E-16));
#12395=CARTESIAN_POINT('Ctrl Pts',(0.297857995688647,1.306435779838,-1.95156391047391E-17));
#12396=CARTESIAN_POINT('Ctrl Pts',(0.289922476296638,1.30625505685688,-1.46278605970555E-13));
#12397=CARTESIAN_POINT('Ctrl Pts',(0.282050301799808,1.30510306275878,-1.25203502999379E-6));
#12398=CARTESIAN_POINT('Ctrl Pts',(0.274405144964298,1.30305953674341,-1.39678564665046E-6));
#12399=CARTESIAN_POINT('Ctrl Pts',(0.269498922713003,1.30174811919849,-1.48967827287246E-6));
#12400=CARTESIAN_POINT('Ctrl Pts',(0.26468600784495,1.30006837070384,-1.17796618578504E-6));
#12401=CARTESIAN_POINT('Ctrl Pts',(0.260012701218123,1.29803054880949,-5.63923085528507E-7));
#12402=CARTESIAN_POINT('Ctrl Pts',(0.252740988282594,1.29485967708789,3.91534262267771E-7));
#12403=CARTESIAN_POINT('Ctrl Pts',(0.245891302634708,1.2908611961912,2.26944434681222E-6));
#12404=CARTESIAN_POINT('Ctrl Pts',(0.239629152465829,1.28609427281,1.73040332626933E-6));
#12405=CARTESIAN_POINT('Ctrl Pts',(0.238677421334952,1.28536978852616,1.6484790500646E-6));
#12406=CARTESIAN_POINT('Ctrl Pts',(0.23773930716971,1.28462746803483,1.50379952206709E-6));
#12407=CARTESIAN_POINT('Ctrl Pts',(0.236815449960777,1.28386742955246,1.27686598471174E-6));
#12408=CARTESIAN_POINT('Ctrl Pts',(0.233849259515119,1.28142720517261,5.48259784756267E-7));
#12409=CARTESIAN_POINT('Ctrl Pts',(0.231029859162728,1.27880446664625,-1.01231737317126E-6));
#12410=CARTESIAN_POINT('Ctrl Pts',(0.228365947504865,1.27601569667724,-2.73789903475208E-6));
#12411=CARTESIAN_POINT('Ctrl Pts',(0.222875659368053,1.2702680771449,-6.2943009513513E-6));
#12412=CARTESIAN_POINT('Ctrl Pts',(0.218108003769119,1.26388547870891,-1.02458913084139E-5));
#12413=CARTESIAN_POINT('Ctrl Pts',(0.214119068651703,1.25703104885628,-1.16727273233865E-5));
#12414=CARTESIAN_POINT('Ctrl Pts',(0.211608035823831,1.25271618840614,-1.25709199407453E-5));
#12415=CARTESIAN_POINT('Ctrl Pts',(0.209406266788438,1.24821342134138,-1.25531979180244E-5));
#12416=CARTESIAN_POINT('Ctrl Pts',(0.207536767894457,1.24355803714115,-1.16467700682383E-5));
#12417=CARTESIAN_POINT('Ctrl Pts',(0.204585779527196,1.23620955211972,-1.02159812889057E-5));
#12418=CARTESIAN_POINT('Ctrl Pts',(0.20249437279756,1.22856635796309,-6.44823334219156E-6));
#12419=CARTESIAN_POINT('Ctrl Pts',(0.201333199355162,1.22077498745768,-3.37414558979738E-6));
#12420=CARTESIAN_POINT('Ctrl Pts',(0.200635497716839,1.21609347152911,-1.5270519663277E-6));
#12421=CARTESIAN_POINT('Ctrl Pts',(0.200274469246579,1.21135795995708,-3.76748562593766E-12));
#12422=CARTESIAN_POINT('Ctrl Pts',(0.200274469199584,1.20659878095028,6.07153216591882E-18));
#12423=CARTESIAN_POINT('',(-2.81723893694256E-19,1.20714678905882,-2.77862675945125E-17));
#12424=CARTESIAN_POINT('',(0.,-1.5,0.));
#12425=CARTESIAN_POINT('',(0.292751161823634,1.50665779898694,0.));
#12426=CARTESIAN_POINT('Ctrl Pts',(0.292751161823634,1.50665779898694,-4.77048955893622E-17));
#12427=CARTESIAN_POINT('Ctrl Pts',(0.274916014309114,1.50625165707847,3.84528327419955E-12));
#12428=CARTESIAN_POINT('Ctrl Pts',(0.257184594685611,1.50420857033458,-2.03607170333744E-6));
#12429=CARTESIAN_POINT('Ctrl Pts',(0.239764500086274,1.50063675387888,-2.79213621391921E-6));
#12430=CARTESIAN_POINT('Ctrl Pts',(0.222116086584643,1.49701812291205,-3.55811018958082E-6));
#12431=CARTESIAN_POINT('Ctrl Pts',(0.204785660682177,1.49183000356027,-2.9511242418033E-6));
#12432=CARTESIAN_POINT('Ctrl Pts',(0.187998620502071,1.4851341555102,-6.80337370794577E-7));
#12433=CARTESIAN_POINT('Ctrl Pts',(0.185044527596802,1.48395585623842,-2.80736529130144E-7));
#12434=CARTESIAN_POINT('Ctrl Pts',(0.182107319868513,1.48273075079643,1.61255976403501E-7));
#12435=CARTESIAN_POINT('Ctrl Pts',(0.17918831289364,1.48145903083089,6.35063889779883E-7));
#12436=CARTESIAN_POINT('Ctrl Pts',(0.162608037952008,1.47423552404966,3.32634402063389E-6));
#12437=CARTESIAN_POINT('Ctrl Pts',(0.146760254055949,1.46557586252388,7.36741945499403E-6));
#12438=CARTESIAN_POINT('Ctrl Pts',(0.131860714325404,1.4555643673366,8.80872142158042E-6));
#12439=CARTESIAN_POINT('Ctrl Pts',(0.12416804976458,1.45039541073654,9.55286874158632E-6));
#12440=CARTESIAN_POINT('Ctrl Pts',(0.116728404005452,1.44486529627202,9.54902993357918E-6));
#12441=CARTESIAN_POINT('Ctrl Pts',(0.109574210210226,1.43898090192647,7.86258910610491E-6));
#12442=CARTESIAN_POINT('Ctrl Pts',(0.100675189791982,1.43166137062374,5.76484451217541E-6));
#12443=CARTESIAN_POINT('Ctrl Pts',(0.0922175942578585,1.42379373777092,
1.07962821494929E-6));
#12444=CARTESIAN_POINT('Ctrl Pts',(0.0842272493232774,1.41542759110015,
-4.17082519724513E-6));
#12445=CARTESIAN_POINT('Ctrl Pts',(0.0719003514327883,1.40252093480537,
-1.22708263387205E-5));
#12446=CARTESIAN_POINT('Ctrl Pts',(0.0607923942774574,1.38854365509349,
-2.1446290640466E-5));
#12447=CARTESIAN_POINT('Ctrl Pts',(0.0509667079859164,1.37370740939602,
-2.73088451608079E-5));
#12448=CARTESIAN_POINT('Ctrl Pts',(0.040988527714452,1.35864090617899,-3.32623861267576E-5));
#12449=CARTESIAN_POINT('Ctrl Pts',(0.0323319291028794,1.34268723517955,
-3.58272570146011E-5));
#12450=CARTESIAN_POINT('Ctrl Pts',(0.0251054147216294,1.32603775378173,
-3.42048160832586E-5));
#12451=CARTESIAN_POINT('Ctrl Pts',(0.0239557673766072,1.32338903116455,
-3.39467061825833E-5));
#12452=CARTESIAN_POINT('Ctrl Pts',(0.022842414085455,1.32072266145131,-3.35898145907185E-5));
#12453=CARTESIAN_POINT('Ctrl Pts',(0.0217659098422027,1.31803938112476,
-3.31388957009043E-5));
#12454=CARTESIAN_POINT('Ctrl Pts',(0.0146851456525434,1.30038996137917,
-3.01729526055095E-5));
#12455=CARTESIAN_POINT('Ctrl Pts',(0.00925910545076598,1.282173175788,-2.28911926108039E-5));
#12456=CARTESIAN_POINT('Ctrl Pts',(0.0055880418397064,1.26361786690427,
-1.53360241296986E-5));
#12457=CARTESIAN_POINT('Ctrl Pts',(0.00217213684284492,1.24635225152695,
-8.30598038733772E-6));
#12458=CARTESIAN_POINT('Ctrl Pts',(0.000275638047107462,1.2287919996398,
-1.11502351997496E-6));
#12459=CARTESIAN_POINT('Ctrl Pts',(2.78020181985954E-5,1.21111091902543,
-1.13803743790751E-7));
#12460=CARTESIAN_POINT('Ctrl Pts',(9.289355304618E-6,1.20979019141994,-3.90154078055202E-8));
#12461=CARTESIAN_POINT('Ctrl Pts',(3.5054796412911E-11,1.20846879032832,
-2.82152417201308E-12));
#12462=CARTESIAN_POINT('Ctrl Pts',(6.5594231435373E-18,1.20714678905882,
2.42861286636753E-17));
#12463=CARTESIAN_POINT('',(12.8678148030684,2.16300527278356,0.));
#12464=CARTESIAN_POINT('Ctrl Pts',(0.292751161823634,1.50665779898694,0.));
#12465=CARTESIAN_POINT('Ctrl Pts',(4.48443904223854,1.60211086545473,0.));
#12466=CARTESIAN_POINT('Ctrl Pts',(8.67612692265345,1.70561506876628,0.));
#12467=CARTESIAN_POINT('Ctrl Pts',(12.8678148030684,2.16300527278356,0.));
#12468=CARTESIAN_POINT('',(13.2,1.86519007666192,1.29914761427265E-16));
#12469=CARTESIAN_POINT('Ctrl Pts',(13.2,1.86519007666192,1.40512601554121E-16));
#12470=CARTESIAN_POINT('Ctrl Pts',(13.2000000013352,1.88296731840607,9.35191444695304E-11));
#12471=CARTESIAN_POINT('Ctrl Pts',(13.1983511006715,1.90064589040826,-4.81925060583158E-6));
#12472=CARTESIAN_POINT('Ctrl Pts',(13.1951709302004,1.91804121845656,-9.22684518112407E-6));
#12473=CARTESIAN_POINT('Ctrl Pts',(13.1919252271695,1.93579500539423,-1.37252653764835E-5));
#12474=CARTESIAN_POINT('Ctrl Pts',(13.1870840836913,1.95325521073227,-1.77396479500911E-5));
#12475=CARTESIAN_POINT('Ctrl Pts',(13.1807207319279,1.9702167899609,-1.88895599539727E-5));
#12476=CARTESIAN_POINT('Ctrl Pts',(13.179605107926,1.97319049715201,-1.90911627380646E-5));
#12477=CARTESIAN_POINT('Ctrl Pts',(13.1784425783122,1.97614882406338,-1.92137058190342E-5));
#12478=CARTESIAN_POINT('Ctrl Pts',(13.1772333926356,1.97909058504493,-1.92562174744009E-5));
#12479=CARTESIAN_POINT('Ctrl Pts',(13.1703491364924,1.99583891121373,-1.94982490583826E-5));
#12480=CARTESIAN_POINT('Ctrl Pts',(13.1620175712498,2.0119031422279,-1.67925698753361E-5));
#12481=CARTESIAN_POINT('Ctrl Pts',(13.1523342210936,2.02708796667103,-1.30402710852334E-5));
#12482=CARTESIAN_POINT('Ctrl Pts',(13.1443502942575,2.03960786168842,-9.94649893779315E-6));
#12483=CARTESIAN_POINT('Ctrl Pts',(13.1354462980072,2.05153020544825,-6.18593217696112E-6));
#12484=CARTESIAN_POINT('Ctrl Pts',(13.1256528604983,2.06273196126272,-4.73977425690188E-6));
#12485=CARTESIAN_POINT('Ctrl Pts',(13.1217453950533,2.06720132901318,-4.16277439392992E-6));
#12486=CARTESIAN_POINT('Ctrl Pts',(13.1176961215346,2.07155579183536,-3.97575052791371E-6));
#12487=CARTESIAN_POINT('Ctrl Pts',(13.1135113749213,2.07579033931164,-3.99023031318383E-6));
#12488=CARTESIAN_POINT('Ctrl Pts',(13.1009362730034,2.08851509208914,-4.03374185458576E-6));
#12489=CARTESIAN_POINT('Ctrl Pts',(13.0872516297578,2.10004749226926,-5.60236028337187E-6));
#12490=CARTESIAN_POINT('Ctrl Pts',(13.0726646436523,2.11028882659185,-6.03124820804926E-6));
#12491=CARTESIAN_POINT('Ctrl Pts',(13.0580194031224,2.12057106059247,-6.46184893473862E-6));
#12492=CARTESIAN_POINT('Ctrl Pts',(13.0424632957183,2.12955278528135,-5.76500392338198E-6));
#12493=CARTESIAN_POINT('Ctrl Pts',(13.0261754841647,2.13709349482706,-4.98347139369932E-6));
#12494=CARTESIAN_POINT('Ctrl Pts',(13.0233759049672,2.13838960594114,-4.84914013593099E-6));
#12495=CARTESIAN_POINT('Ctrl Pts',(13.0205546633935,2.13964302898522,-4.72077764982159E-6));
#12496=CARTESIAN_POINT('Ctrl Pts',(13.0177126224567,2.14085289970554,-4.61407510358037E-6));
#12497=CARTESIAN_POINT('Ctrl Pts',(13.0148367726024,2.14207716304734,-4.50610322390289E-6));
#12498=CARTESIAN_POINT('Ctrl Pts',(13.0119432782921,2.14325527660784,-4.42172619954107E-6));
#12499=CARTESIAN_POINT('Ctrl Pts',(13.0090331608036,2.14438664763146,-4.38057543634576E-6));
#12500=CARTESIAN_POINT('Ctrl Pts',(12.9922536897216,2.1509100294015,-4.14330390220891E-6));
#12501=CARTESIAN_POINT('Ctrl Pts',(12.9749229882599,2.15588345271621,-5.05640020348117E-6));
#12502=CARTESIAN_POINT('Ctrl Pts',(12.9572550825995,2.15928949382789,-4.85686529648217E-6));
#12503=CARTESIAN_POINT('Ctrl Pts',(12.9529252316797,2.16012420794307,-4.80796553341985E-6));
#12504=CARTESIAN_POINT('Ctrl Pts',(12.9485750628159,2.16086455090717,-4.70814629363608E-6));
#12505=CARTESIAN_POINT('Ctrl Pts',(12.944207640703,2.16150979950679,-4.55317442353944E-6));
#12506=CARTESIAN_POINT('Ctrl Pts',(12.9263774359968,2.16414405704371,-3.92049452767182E-6));
#12507=CARTESIAN_POINT('Ctrl Pts',(12.9083632163621,2.16518216214944,-2.15504024707585E-6));
#12508=CARTESIAN_POINT('Ctrl Pts',(12.8903762705535,2.16459816844574,-9.12104093693782E-7));
#12509=CARTESIAN_POINT('Ctrl Pts',(12.8828459063217,2.16435367528137,-3.91739933400607E-7));
#12510=CARTESIAN_POINT('Ctrl Pts',(12.8753202361859,2.1638242536466,5.87463683432524E-12));
#12511=CARTESIAN_POINT('Ctrl Pts',(12.8678148030684,2.16300527278357,2.8796409701215E-16));
#12512=CARTESIAN_POINT('',(13.2,-1.86519007666192,1.11326398357188E-16));
#12513=CARTESIAN_POINT('',(13.2,2.2,0.));
#12514=CARTESIAN_POINT('',(12.8678148030684,-2.16300527278356,1.38777878078145E-17));
#12515=CARTESIAN_POINT('Ctrl Pts',(12.8678148030684,-2.16300527278357,2.56739074444567E-16));
#12516=CARTESIAN_POINT('Ctrl Pts',(12.8854929372559,-2.16493428409685,8.24591542686399E-11));
#12517=CARTESIAN_POINT('Ctrl Pts',(12.9032520674897,-2.16521372082443,-4.52295339524789E-6));
#12518=CARTESIAN_POINT('Ctrl Pts',(12.9208958607904,-2.1639404182545,-8.68231213275745E-6));
#12519=CARTESIAN_POINT('Ctrl Pts',(12.9389012534027,-2.16264102008682,-1.29269145154966E-5));
#12520=CARTESIAN_POINT('Ctrl Pts',(12.9567880250381,-2.15972433317902,-1.67278855193166E-5));
#12521=CARTESIAN_POINT('Ctrl Pts',(12.9743443410528,-2.15524079327399,-1.78237954457702E-5));
#12522=CARTESIAN_POINT('Ctrl Pts',(12.9774431846623,-2.15444940919484,-1.80172331504298E-5));
#12523=CARTESIAN_POINT('Ctrl Pts',(12.9805316913262,-2.15360908525727,-1.81351031595367E-5));
#12524=CARTESIAN_POINT('Ctrl Pts',(12.9836086301392,-2.15271994254544,-1.81766625580856E-5));
#12525=CARTESIAN_POINT('Ctrl Pts',(13.0010041030966,-2.14769317440371,-1.84116186093898E-5));
#12526=CARTESIAN_POINT('Ctrl Pts',(13.017876958431,-2.14115457229109,-1.5854618169158E-5));
#12527=CARTESIAN_POINT('Ctrl Pts',(13.0340226638693,-2.13317744288338,-1.23136839993165E-5));
#12528=CARTESIAN_POINT('Ctrl Pts',(13.0473215411186,-2.12660684953271,-9.39709115965876E-6));
#12529=CARTESIAN_POINT('Ctrl Pts',(13.060127470267,-2.11905920305061,-5.85016632862467E-6));
#12530=CARTESIAN_POINT('Ctrl Pts',(13.0723151314263,-2.11055132433008,-4.53327195050794E-6));
#12531=CARTESIAN_POINT('Ctrl Pts',(13.0772147086919,-2.10713106111368,-4.00386555564548E-6));
#12532=CARTESIAN_POINT('Ctrl Pts',(13.0820141951123,-2.10355537352593,-3.85636210984559E-6));
#12533=CARTESIAN_POINT('Ctrl Pts',(13.0867078006727,-2.0998301147952,-3.90248451975241E-6));
#12534=CARTESIAN_POINT('Ctrl Pts',(13.1007249787291,-2.08870484782034,-4.04022639510273E-6));
#12535=CARTESIAN_POINT('Ctrl Pts',(13.1136765748478,-2.07634683247102,-5.5945154994439E-6));
#12536=CARTESIAN_POINT('Ctrl Pts',(13.1254414850725,-2.06295113861397,-5.97495381195624E-6));
#12537=CARTESIAN_POINT('Ctrl Pts',(13.1372476314214,-2.04950849272046,-6.35672556443159E-6));
#12538=CARTESIAN_POINT('Ctrl Pts',(13.1478597809499,-2.03501968083851,-5.56609061204695E-6));
#12539=CARTESIAN_POINT('Ctrl Pts',(13.1571184147632,-2.01964723728874,-4.75455255839871E-6));
#12540=CARTESIAN_POINT('Ctrl Pts',(13.158708901902,-2.01700649414547,-4.61514313115074E-6));
#12541=CARTESIAN_POINT('Ctrl Pts',(13.1602593369672,-2.01433961799121,-4.48389992381974E-6));
#12542=CARTESIAN_POINT('Ctrl Pts',(13.1617687665475,-2.01164737048868,-4.37752847101542E-6));
#12543=CARTESIAN_POINT('Ctrl Pts',(13.1632768494098,-2.00895752501823,-4.27125192317111E-6));
#12544=CARTESIAN_POINT('Ctrl Pts',(13.164742106841,-2.00624572954308,-4.19089851494128E-6));
#12545=CARTESIAN_POINT('Ctrl Pts',(13.1661638648313,-2.00351289682408,-4.15637526360595E-6));
#12546=CARTESIAN_POINT('Ctrl Pts',(13.1744716670281,-1.98754405133797,-3.95464448717833E-6));
#12547=CARTESIAN_POINT('Ctrl Pts',(13.181298057795,-1.97085874357403,-5.01850453361653E-6));
#12548=CARTESIAN_POINT('Ctrl Pts',(13.1866022393826,-1.95366776591112,-4.89891140766866E-6));
#12549=CARTESIAN_POINT('Ctrl Pts',(13.1879075264936,-1.94943729958961,-4.86948116225E-6));
#12550=CARTESIAN_POINT('Ctrl Pts',(13.1891204013114,-1.94517611908519,-4.78523710928743E-6));
#12551=CARTESIAN_POINT('Ctrl Pts',(13.1902397948733,-1.94088722910442,-4.64104147683466E-6));
#12552=CARTESIAN_POINT('Ctrl Pts',(13.1947901580114,-1.92345278286841,-4.05488258426869E-6));
#12553=CARTESIAN_POINT('Ctrl Pts',(13.1977733658442,-1.90566244769967,-2.24449026644408E-6));
#12554=CARTESIAN_POINT('Ctrl Pts',(13.1991406030032,-1.88772335428786,-9.50757284845071E-7));
#12555=CARTESIAN_POINT('Ctrl Pts',(13.1997114533543,-1.8802334044254,-4.10596478211383E-7));
#12556=CARTESIAN_POINT('Ctrl Pts',(13.2000000000958,-1.87271737110067,6.9401096738129E-12));
#12557=CARTESIAN_POINT('Ctrl Pts',(13.2,-1.86519007666192,1.81278603239576E-16));
#12558=CARTESIAN_POINT('',(0.292751161823634,-1.50665779898694,-1.38777878078145E-17));
#12559=CARTESIAN_POINT('Ctrl Pts',(12.8678148030684,-2.16300527278356,0.));
#12560=CARTESIAN_POINT('Ctrl Pts',(8.67612692265345,-1.70561506876628,0.));
#12561=CARTESIAN_POINT('Ctrl Pts',(4.48443904223854,-1.60211086545473,0.));
#12562=CARTESIAN_POINT('Ctrl Pts',(0.292751161823634,-1.50665779898694,
0.));
#12563=CARTESIAN_POINT('',(4.02814324098787E-18,-1.20714678905882,5.54818711994559E-17));
#12564=CARTESIAN_POINT('Ctrl Pts',(-2.22044604925031E-16,-1.20714678905882,
-3.98986399474666E-17));
#12565=CARTESIAN_POINT('Ctrl Pts',(2.12382277713531E-10,-1.2249878157372,
-1.35440422383976E-12));
#12566=CARTESIAN_POINT('Ctrl Pts',(0.00163882612763064,-1.24276245549475,
-1.96699749426327E-6));
#12567=CARTESIAN_POINT('Ctrl Pts',(0.00481304415265273,-1.26026068126938,
-2.66007142975038E-6));
#12568=CARTESIAN_POINT('Ctrl Pts',(0.00802873944670128,-1.27798755504872,
-3.36220171040687E-6));
#12569=CARTESIAN_POINT('Ctrl Pts',(0.0128206026099745,-1.29543230475431,
-2.69550948014298E-6));
#12570=CARTESIAN_POINT('Ctrl Pts',(0.0191320595672371,-1.31236817798419,
-4.00401478067381E-7));
#12571=CARTESIAN_POINT('Ctrl Pts',(0.0202443702650641,-1.31535290133701,
4.0809101773195E-9));
#12572=CARTESIAN_POINT('Ctrl Pts',(0.0214039964883031,-1.3183217636574,
4.5005107558061E-7));
#12573=CARTESIAN_POINT('Ctrl Pts',(0.0226107760969305,-1.32127343934773,
9.26779280916758E-7));
#12574=CARTESIAN_POINT('Ctrl Pts',(0.0294548697216842,-1.33801348419941,
3.63048130534217E-6));
#12575=CARTESIAN_POINT('Ctrl Pts',(0.0377511831708778,-1.35405403406083,
7.64722139837078E-6));
#12576=CARTESIAN_POINT('Ctrl Pts',(0.0474204318104353,-1.36917746582299,
9.03443059383348E-6));
#12577=CARTESIAN_POINT('Ctrl Pts',(0.0524109755304394,-1.37698305136733,
9.75040433665629E-6));
#12578=CARTESIAN_POINT('Ctrl Pts',(0.0577680562174045,-1.38454410063597,
9.71159147480002E-6));
#12579=CARTESIAN_POINT('Ctrl Pts',(0.0634855547170043,-1.39182806229354,
7.98761394269614E-6));
#12580=CARTESIAN_POINT('Ctrl Pts',(0.0706048733905122,-1.40089791062835,
5.84095042579577E-6));
#12581=CARTESIAN_POINT('Ctrl Pts',(0.0782829434694699,-1.40953838460506,
1.09773645972912E-6));
#12582=CARTESIAN_POINT('Ctrl Pts',(0.0864706998703675,-1.41772246232928,
-4.21049985396393E-6));
#12583=CARTESIAN_POINT('Ctrl Pts',(0.0990944981487371,-1.43034058886193,
-1.2394683793612E-5));
#12584=CARTESIAN_POINT('Ctrl Pts',(0.112816484288725,-1.44176429483685,
-2.16481703631134E-5));
#12585=CARTESIAN_POINT('Ctrl Pts',(0.127426518150943,-1.45192534842919,
-2.7562374581111E-5));
#12586=CARTESIAN_POINT('Ctrl Pts',(0.142261949549145,-1.46224316253723,
-3.35678206860622E-5));
#12587=CARTESIAN_POINT('Ctrl Pts',(0.158014355623482,-1.47125989363127,
-3.6155642403295E-5));
#12588=CARTESIAN_POINT('Ctrl Pts',(0.17449494651519,-1.47886261331763,-3.45187637154371E-5));
#12589=CARTESIAN_POINT('Ctrl Pts',(0.177115379630184,-1.48007145458801,
-3.42584981007467E-5));
#12590=CARTESIAN_POINT('Ctrl Pts',(0.179754261386328,-1.48124444832217,
-3.38986806574493E-5));
#12591=CARTESIAN_POINT('Ctrl Pts',(0.18241086941249,-1.48238102342202,-3.34441145409493E-5));
#12592=CARTESIAN_POINT('Ctrl Pts',(0.199890279181845,-1.48985922935543,
-3.04532527580594E-5));
#12593=CARTESIAN_POINT('Ctrl Pts',(0.217974246898519,-1.49569663469242,
-2.31073027206853E-5));
#12594=CARTESIAN_POINT('Ctrl Pts',(0.236436446036386,-1.49978781870256,
-1.54828395726751E-5));
#12595=CARTESIAN_POINT('Ctrl Pts',(0.253618559172887,-1.50359533838099,
-8.38702246898572E-6));
#12596=CARTESIAN_POINT('Ctrl Pts',(0.271129804961754,-1.50589051664322,
-1.1237837803371E-6));
#12597=CARTESIAN_POINT('Ctrl Pts',(0.288799387895208,-1.50654014509364,
-1.14426782679271E-7));
#12598=CARTESIAN_POINT('Ctrl Pts',(0.290115790923368,-1.5065885431154,-3.92285953074499E-8));
#12599=CARTESIAN_POINT('Ctrl Pts',(0.291433072638222,-1.50662778343727,
-2.32210426557352E-12));
#12600=CARTESIAN_POINT('Ctrl Pts',(0.292751161823634,-1.50665779898694,
2.86229373536173E-17));
#12601=CARTESIAN_POINT('',(0.,-1.5,0.));
#12602=CARTESIAN_POINT('',(0.297857995688647,-1.306435779838,0.));
#12603=CARTESIAN_POINT('Ctrl Pts',(0.200274469199585,-1.20659878095028,
-5.63785129692462E-18));
#12604=CARTESIAN_POINT('Ctrl Pts',(0.200274469233139,-1.21453676310593,
-8.71436967499621E-13));
#12605=CARTESIAN_POINT('Ctrl Pts',(0.201246859971722,-1.22243356087926,
-1.21395871814677E-6));
#12606=CARTESIAN_POINT('Ctrl Pts',(0.203115675186186,-1.23012372049816,
-1.3343733317444E-6));
#12607=CARTESIAN_POINT('Ctrl Pts',(0.204315340901654,-1.23506033529553,
-1.41167219064517E-6));
#12608=CARTESIAN_POINT('Ctrl Pts',(0.20588557457721,-1.23991201018842,-1.08820351238587E-6));
#12609=CARTESIAN_POINT('Ctrl Pts',(0.207817175189242,-1.24463217458037,
-4.7123943162984E-7));
#12610=CARTESIAN_POINT('Ctrl Pts',(0.210821635148072,-1.25197403646754,
4.8840194822981E-7));
#12611=CARTESIAN_POINT('Ctrl Pts',(0.214662962735955,-1.25891288736431,
2.34840446672759E-6));
#12612=CARTESIAN_POINT('Ctrl Pts',(0.219285851586231,-1.26528190572196,
1.77850405974346E-6));
#12613=CARTESIAN_POINT('Ctrl Pts',(0.219987799701267,-1.26624898941694,
1.69196931287913E-6));
#12614=CARTESIAN_POINT('Ctrl Pts',(0.220707854727247,-1.26720289123473,
1.54254180957111E-6));
#12615=CARTESIAN_POINT('Ctrl Pts',(0.221445913570039,-1.26814297034805,
1.31084431541716E-6));
#12616=CARTESIAN_POINT('Ctrl Pts',(0.223819423285066,-1.27116615329633,
5.65732650279818E-7));
#12617=CARTESIAN_POINT('Ctrl Pts',(0.226378993511503,-1.27404655624932,
-1.0141799309673E-6));
#12618=CARTESIAN_POINT('Ctrl Pts',(0.229108317341547,-1.27677508245113,
-2.75886047820546E-6));
#12619=CARTESIAN_POINT('Ctrl Pts',(0.234729699316268,-1.28239482161129,
-6.35224711555937E-6));
#12620=CARTESIAN_POINT('Ctrl Pts',(0.241002345945823,-1.28730653457646,
-1.03364935932408E-5));
#12621=CARTESIAN_POINT('Ctrl Pts',(0.247764463424355,-1.29145035967733,
-1.17765252099068E-5));
#12622=CARTESIAN_POINT('Ctrl Pts',(0.25202072563572,-1.29405859685204,-1.26829206064147E-5));
#12623=CARTESIAN_POINT('Ctrl Pts',(0.25647185453211,-1.29636195369988,-1.26655904667795E-5));
#12624=CARTESIAN_POINT('Ctrl Pts',(0.261083107941716,-1.29833661269995,
-1.17517412599227E-5));
#12625=CARTESIAN_POINT('Ctrl Pts',(0.268362152520619,-1.30145368947124,
-1.0309194402435E-5));
#12626=CARTESIAN_POINT('Ctrl Pts',(0.275955349537693,-1.30371808689536,
-6.50743389458559E-6));
#12627=CARTESIAN_POINT('Ctrl Pts',(0.283717840216357,-1.30505580179168,
-3.40467605837577E-6));
#12628=CARTESIAN_POINT('Ctrl Pts',(0.288379557365255,-1.3058591584372,-1.54133347766382E-6));
#12629=CARTESIAN_POINT('Ctrl Pts',(0.293102847896135,-1.30632748638856,
-3.09915230996644E-12));
#12630=CARTESIAN_POINT('Ctrl Pts',(0.297857995688647,-1.306435779838,2.90566182226115E-17));
#12631=CARTESIAN_POINT('',(0.9,-1.32024227787037,0.));
#12632=CARTESIAN_POINT('Ctrl Pts',(0.297857995688651,-1.306435779838,-5.81335652359571E-17));
#12633=CARTESIAN_POINT('Ctrl Pts',(0.498765834064439,-1.31101124067384,
-1.02216845336465E-13));
#12634=CARTESIAN_POINT('Ctrl Pts',(0.699470314209512,-1.31560060357718,
-4.73070532165219E-10));
#12635=CARTESIAN_POINT('Ctrl Pts',(0.9,-1.32024227787037,4.62320796019307E-17));
#12636=CARTESIAN_POINT('',(0.9,1.39290118819044,0.));
#12637=CARTESIAN_POINT('',(4.3,-1.41116952203211,0.));
#12638=CARTESIAN_POINT('Ctrl Pts',(1.10000000020724,-1.32489175811528,-9.82782277325449E-12));
#12639=CARTESIAN_POINT('Ctrl Pts',(2.16992692797068,-1.34987955410658,4.63225598025733E-9));
#12640=CARTESIAN_POINT('Ctrl Pts',(3.23514201430925,-1.37672428034078,3.20747301048384E-8));
#12641=CARTESIAN_POINT('Ctrl Pts',(4.3,-1.41116952203211,-8.74629427996717E-16));
#12642=CARTESIAN_POINT('',(4.3,1.48481481481482,0.));
#12643=CARTESIAN_POINT('',(8.7,-1.61160179736194,0.));
#12644=CARTESIAN_POINT('Ctrl Pts',(4.50000000001737,-1.41772989873549,-1.00870158580013E-12));
#12645=CARTESIAN_POINT('Ctrl Pts',(5.14541122039116,-1.43919849219739,1.84287460122322E-8));
#12646=CARTESIAN_POINT('Ctrl Pts',(5.79079200637672,-1.46358894290692,-2.29215846350395E-9));
#12647=CARTESIAN_POINT('Ctrl Pts',(6.43711407552466,-1.49221504703413,-7.12038357450289E-9));
#12648=CARTESIAN_POINT('Ctrl Pts',(6.48784335049204,-1.49446188584227,-7.49934689782436E-9));
#12649=CARTESIAN_POINT('Ctrl Pts',(6.5385784252675,-1.49673484630497,-7.6873350528488E-9));
#12650=CARTESIAN_POINT('Ctrl Pts',(6.58931977021612,-1.49903457911226,-7.60400982311631E-9));
#12651=CARTESIAN_POINT('Ctrl Pts',(7.29382172663923,-1.5309644828944,-6.44710735180711E-9));
#12652=CARTESIAN_POINT('Ctrl Pts',(7.99729122590638,-1.56795478022256,5.29179522587699E-9));
#12653=CARTESIAN_POINT('Ctrl Pts',(8.70000000002062,-1.61160179731554,-3.21479112539667E-13));
#12654=CARTESIAN_POINT('',(8.7,1.68851851851852,0.));
#12655=CARTESIAN_POINT('',(12.6,-1.93292824674167,0.));
#12656=CARTESIAN_POINT('',(12.8889963716306,-1.96391015057091,0.));
#12657=CARTESIAN_POINT('Ctrl Pts',(12.6000000004653,-1.93292824679067,-1.00288700954909E-16));
#12658=CARTESIAN_POINT('Ctrl Pts',(12.6963367945484,-1.94307238002033,2.28133307867826E-10));
#12659=CARTESIAN_POINT('Ctrl Pts',(12.7926686848896,-1.9533982851754,-5.07154825701885E-13));
#12660=CARTESIAN_POINT('Ctrl Pts',(12.8889963716306,-1.96391015057091,2.24786696790336E-16));
#12661=CARTESIAN_POINT('',(12.9997255308004,-1.86463850151065,-1.38777878078145E-17));
#12662=CARTESIAN_POINT('Ctrl Pts',(12.8889963716306,-1.96391015057091,5.29090660172926E-17));
#12663=CARTESIAN_POINT('Ctrl Pts',(12.8968843421745,-1.96477093437063,1.28387508960266E-11));
#12664=CARTESIAN_POINT('Ctrl Pts',(12.9048206871516,-1.96464841285931,-2.5989605143924E-6));
#12665=CARTESIAN_POINT('Ctrl Pts',(12.9126487282508,-1.9636130141884,-4.24292438262167E-6));
#12666=CARTESIAN_POINT('Ctrl Pts',(12.9176900487482,-1.96294620923983,-5.30165014054907E-6));
#12667=CARTESIAN_POINT('Ctrl Pts',(12.9226867577298,-1.96189962975099,-6.00943773338864E-6));
#12668=CARTESIAN_POINT('Ctrl Pts',(12.9275953864907,-1.96048085896027,-6.09358828708331E-6));
#12669=CARTESIAN_POINT('Ctrl Pts',(12.9352257743335,-1.95827540160737,-6.22439902734509E-6));
#12670=CARTESIAN_POINT('Ctrl Pts',(12.9425549137553,-1.95519874430406,-4.64402662178521E-6));
#12671=CARTESIAN_POINT('Ctrl Pts',(12.949425376669,-1.9513005478593,-3.15156624759025E-6));
#12672=CARTESIAN_POINT('Ctrl Pts',(12.9520760960011,-1.94979656991686,-2.57575445499556E-6));
#12673=CARTESIAN_POINT('Ctrl Pts',(12.9546583803074,-1.94816978416017,-2.04880625960079E-6));
#12674=CARTESIAN_POINT('Ctrl Pts',(12.9571622133441,-1.9464211898676,-1.82278374303809E-6));
#12675=CARTESIAN_POINT('Ctrl Pts',(12.9587955877505,-1.9452804951316,-1.67533805140214E-6));
#12676=CARTESIAN_POINT('Ctrl Pts',(12.9603955609302,-1.94408794089591,-1.65796127395168E-6));
#12677=CARTESIAN_POINT('Ctrl Pts',(12.9619602112942,-1.94284549575182,-1.70649031798611E-6));
#12678=CARTESIAN_POINT('Ctrl Pts',(12.9681665721336,-1.93791719798967,-1.89898620422551E-6));
#12679=CARTESIAN_POINT('Ctrl Pts',(12.9737470546445,-1.93226498850035,-2.8025064238469E-6));
#12680=CARTESIAN_POINT('Ctrl Pts',(12.9786034821464,-1.926037248212,-2.79230211737029E-6));
#12681=CARTESIAN_POINT('Ctrl Pts',(12.9817011960737,-1.92206483066456,-2.78579321297956E-6));
#12682=CARTESIAN_POINT('Ctrl Pts',(12.9845038017717,-1.91785723501915,-2.48811564693169E-6));
#12683=CARTESIAN_POINT('Ctrl Pts',(12.9869771252785,-1.91344616543364,-2.2918341012218E-6));
#12684=CARTESIAN_POINT('Ctrl Pts',(12.9874796596041,-1.91254991636901,-2.25195326317628E-6));
#12685=CARTESIAN_POINT('Ctrl Pts',(12.9879679417815,-1.9116463809131,-2.21866365029432E-6));
#12686=CARTESIAN_POINT('Ctrl Pts',(12.98844174868,-1.91073586520696,-2.19841011183313E-6));
#12687=CARTESIAN_POINT('Ctrl Pts',(12.9918929665356,-1.9041036526468,-2.05088297829219E-6));
#12688=CARTESIAN_POINT('Ctrl Pts',(12.9945793344589,-1.89710244289626,-2.35789128083535E-6));
#12689=CARTESIAN_POINT('Ctrl Pts',(12.9964698429198,-1.88986530397042,-1.93853625224654E-6));
#12690=CARTESIAN_POINT('Ctrl Pts',(12.9984668213505,-1.88222058265133,-1.49556391743615E-6));
#12691=CARTESIAN_POINT('Ctrl Pts',(12.9995610814633,-1.87437060764114,-2.4459616079733E-7));
#12692=CARTESIAN_POINT('Ctrl Pts',(12.9997084424383,-1.86646992060833,-2.60951667192209E-8));
#12693=CARTESIAN_POINT('Ctrl Pts',(12.9997198235207,-1.86585972940924,-9.21975031242219E-9));
#12694=CARTESIAN_POINT('Ctrl Pts',(12.9997255308031,-1.86524923282631,2.14479566203628E-13));
#12695=CARTESIAN_POINT('Ctrl Pts',(12.9997255308004,-1.86463850151065,-9.54097911787244E-18));
#12696=CARTESIAN_POINT('',(12.9997255308004,1.86463850151064,1.38777878078145E-17));
#12697=CARTESIAN_POINT('',(12.9997255308004,1.1,0.));
#12698=CARTESIAN_POINT('',(12.8889963716306,1.96391015057091,0.));
#12699=CARTESIAN_POINT('Ctrl Pts',(12.9997255308004,1.86463850151065,-9.97465998686664E-18));
#12700=CARTESIAN_POINT('Ctrl Pts',(12.9997255309996,1.87257112921612,1.42345874390777E-11));
#12701=CARTESIAN_POINT('Ctrl Pts',(12.9987425107347,1.88044501776258,-2.76622459581243E-6));
#12702=CARTESIAN_POINT('Ctrl Pts',(12.9968635501128,1.8881121101061,-4.50602169498049E-6));
#12703=CARTESIAN_POINT('Ctrl Pts',(12.9956551765012,1.89304287446485,-5.62489820561454E-6));
#12704=CARTESIAN_POINT('Ctrl Pts',(12.994075066483,1.89788828888188,-6.37205869803057E-6));
#12705=CARTESIAN_POINT('Ctrl Pts',(12.9921354490207,1.90260616696402,-6.45954116508302E-6));
#12706=CARTESIAN_POINT('Ctrl Pts',(12.9891151690915,1.90995262200289,-6.59576469602218E-6));
#12707=CARTESIAN_POINT('Ctrl Pts',(12.9852608829945,1.91690476599405,-4.92589918404109E-6));
#12708=CARTESIAN_POINT('Ctrl Pts',(12.9806393828366,1.92331154882078,-3.3382766296878E-6));
#12709=CARTESIAN_POINT('Ctrl Pts',(12.9788533632605,1.92578750666072,-2.72472586378502E-6));
#12710=CARTESIAN_POINT('Ctrl Pts',(12.9769522584487,1.92818179997524,-2.1610482659023E-6));
#12711=CARTESIAN_POINT('Ctrl Pts',(12.9749381758772,1.93048453804291,-1.90960564360578E-6));
#12712=CARTESIAN_POINT('Ctrl Pts',(12.9736352090466,1.93197424425657,-1.74694031832382E-6));
#12713=CARTESIAN_POINT('Ctrl Pts',(12.9722849384098,1.93342561524533,-1.71698229815602E-6));
#12714=CARTESIAN_POINT('Ctrl Pts',(12.9708894910408,1.9348369915754,-1.75552529092739E-6));
#12715=CARTESIAN_POINT('Ctrl Pts',(12.9653179015399,1.94047218048862,-1.90941553332435E-6));
#12716=CARTESIAN_POINT('Ctrl Pts',(12.9590944588136,1.94540670303376,-2.83773366290493E-6));
#12717=CARTESIAN_POINT('Ctrl Pts',(12.9523775255978,1.94955941520082,-2.8574013135715E-6));
#12718=CARTESIAN_POINT('Ctrl Pts',(12.9480923984168,1.95220867479748,-2.86994846593266E-6));
#12719=CARTESIAN_POINT('Ctrl Pts',(12.9436054681019,1.95453912223498,-2.59559485065602E-6));
#12720=CARTESIAN_POINT('Ctrl Pts',(12.9389519978263,1.95652032281755,-2.39773084743613E-6));
#12721=CARTESIAN_POINT('Ctrl Pts',(12.9379934875219,1.95692840561619,-2.35697530915642E-6));
#12722=CARTESIAN_POINT('Ctrl Pts',(12.9370291206935,1.95732112306527,-2.32193094846859E-6));
#12723=CARTESIAN_POINT('Ctrl Pts',(12.9360592398442,1.95769827921557,-2.29894501965994E-6));
#12724=CARTESIAN_POINT('Ctrl Pts',(12.929096105975,1.96040602292032,-2.13392052256244E-6));
#12725=CARTESIAN_POINT('Ctrl Pts',(12.9218497638689,1.96231496375013,-2.36509085467933E-6));
#12726=CARTESIAN_POINT('Ctrl Pts',(12.9144555496645,1.96340894166242,-1.92146179377921E-6));
#12727=CARTESIAN_POINT('Ctrl Pts',(12.9066371708262,1.96456567495722,-1.45238421961943E-6));
#12728=CARTESIAN_POINT('Ctrl Pts',(12.8987125532455,1.96480297730229,-2.37321368026999E-7));
#12729=CARTESIAN_POINT('Ctrl Pts',(12.8908401755085,1.96409377829808,-2.55627471131237E-8));
#12730=CARTESIAN_POINT('Ctrl Pts',(12.89022523009,1.96403837970149,-9.02136684357828E-9));
#12731=CARTESIAN_POINT('Ctrl Pts',(12.8896106033158,1.96397717928728,1.9621770460073E-13));
#12732=CARTESIAN_POINT('Ctrl Pts',(12.8889963716306,1.96391015057091,-3.29597460435593E-17));
#12733=CARTESIAN_POINT('',(12.6,1.93292824674167,0.));
#12734=CARTESIAN_POINT('Ctrl Pts',(12.8889963716306,1.96391015057091,8.95144418658345E-17));
#12735=CARTESIAN_POINT('Ctrl Pts',(12.7926686852738,1.95339828521733,-5.07275478770449E-13));
#12736=CARTESIAN_POINT('Ctrl Pts',(12.6963367949308,1.94307238006059,2.28132759158623E-10));
#12737=CARTESIAN_POINT('Ctrl Pts',(12.6000000004652,1.93292824679066,-1.5019386425618E-16));
#12738=CARTESIAN_POINT('',(12.6,-1.99376954809806,0.));
#12739=CARTESIAN_POINT('Origin',(11.2,0.,0.));
#12740=CARTESIAN_POINT('',(10.8,-4.89858719658942E-17,0.7));
#12741=CARTESIAN_POINT('Origin',(11.2,0.,0.7));
#12742=CARTESIAN_POINT('',(10.8,-4.89858719658942E-17,0.));
#12743=CARTESIAN_POINT('Origin',(2.,0.,0.));
#12744=CARTESIAN_POINT('',(1.6,-4.89858719658941E-17,0.));
#12745=CARTESIAN_POINT('Origin',(12.6,-1.99376954809806,0.));
#12746=CARTESIAN_POINT('',(12.6,-1.90428042248893,0.60470250816874));
#12747=CARTESIAN_POINT('Ctrl Pts',(12.6,-1.93292824674167,0.));
#12748=CARTESIAN_POINT('Ctrl Pts',(12.6,-1.92814118331811,0.100975624959503));
#12749=CARTESIAN_POINT('Ctrl Pts',(12.6,-1.9233557423333,0.20195205683881));
#12750=CARTESIAN_POINT('Ctrl Pts',(12.6,-1.91380649287245,0.40351907263528));
#12751=CARTESIAN_POINT('Ctrl Pts',(12.6,-1.90904260275794,0.504111110768618));
#12752=CARTESIAN_POINT('Ctrl Pts',(12.6,-1.90428042248893,0.60470250816874));
#12753=CARTESIAN_POINT('',(12.6,1.90428042248893,0.60470250816874));
#12754=CARTESIAN_POINT('Ctrl Pts',(12.6,1.90428042248893,0.60470250816874));
#12755=CARTESIAN_POINT('Ctrl Pts',(12.6,1.90904310126474,0.504100580823831));
#12756=CARTESIAN_POINT('Ctrl Pts',(12.6,1.91380749024866,0.403498012513773));
#12757=CARTESIAN_POINT('Ctrl Pts',(12.6,1.92335674041114,0.201930996640285));
#12758=CARTESIAN_POINT('Ctrl Pts',(12.6,1.92814168252712,0.100965094925255));
#12759=CARTESIAN_POINT('Ctrl Pts',(12.6,1.93292824674167,0.));
#12760=CARTESIAN_POINT('',(12.6,1.80383022254432,0.7));
#12761=CARTESIAN_POINT('Ctrl Pts',(12.6,1.80383022254432,0.7));
#12762=CARTESIAN_POINT('Ctrl Pts',(12.6,1.81177675668304,0.7));
#12763=CARTESIAN_POINT('Ctrl Pts',(12.6000021803669,1.81966206665253,0.699006623620781));
#12764=CARTESIAN_POINT('Ctrl Pts',(12.6000040789681,1.8273451885609,0.69711902809518));
#12765=CARTESIAN_POINT('Ctrl Pts',(12.6000050614635,1.8313210797205,0.696142227980247));
#12766=CARTESIAN_POINT('Ctrl Pts',(12.6000059683507,1.83524283435206,0.694925046992878));
#12767=CARTESIAN_POINT('Ctrl Pts',(12.6000066021136,1.83908960013903,0.693475985595303));
#12768=CARTESIAN_POINT('Ctrl Pts',(12.6000078338507,1.84656590463324,0.690659691378536));
#12769=CARTESIAN_POINT('Ctrl Pts',(12.6000078244032,1.85367932786264,0.687000939374075));
#12770=CARTESIAN_POINT('Ctrl Pts',(12.6000065509639,1.86028396908448,0.682580904467878));
#12771=CARTESIAN_POINT('Ctrl Pts',(12.600005740321,1.86448833536622,0.679767209507086));
#12772=CARTESIAN_POINT('Ctrl Pts',(12.6000044390918,1.86848632867783,0.676643963831362));
#12773=CARTESIAN_POINT('Ctrl Pts',(12.6000033339006,1.8722338275817,0.673223162566374));
#12774=CARTESIAN_POINT('Ctrl Pts',(12.6000024442799,1.87525036668517,0.670469597843409));
#12775=CARTESIAN_POINT('Ctrl Pts',(12.600001679327,1.8780865799519,0.667539409933064));
#12776=CARTESIAN_POINT('Ctrl Pts',(12.600001676908,1.88072259809992,0.664442334323256));
#12777=CARTESIAN_POINT('Ctrl Pts',(12.6000016722164,1.88583495965423,0.658435786041233));
#12778=CARTESIAN_POINT('Ctrl Pts',(12.6000042182276,1.89019731592974,0.651802923597933));
#12779=CARTESIAN_POINT('Ctrl Pts',(12.6000050838539,1.89374834224248,0.644708005294394));
#12780=CARTESIAN_POINT('Ctrl Pts',(12.60000518898,1.89417959722901,0.643846361750254));
#12781=CARTESIAN_POINT('Ctrl Pts',(12.6000052753339,1.8945988291305,0.642977876839351));
#12782=CARTESIAN_POINT('Ctrl Pts',(12.6000053405091,1.89500587920016,0.642102827114796));
#12783=CARTESIAN_POINT('Ctrl Pts',(12.6000058761205,1.89835102950234,0.634911640898031));
#12784=CARTESIAN_POINT('Ctrl Pts',(12.6000044960414,1.90083797337412,0.627363460372113));
#12785=CARTESIAN_POINT('Ctrl Pts',(12.6000025707297,1.90241244660326,0.619625605651968));
#12786=CARTESIAN_POINT('Ctrl Pts',(12.6000013488022,1.90341170938816,0.614714661398562));
#12787=CARTESIAN_POINT('Ctrl Pts',(12.5999999979477,1.90404256918024,0.609726685483646));
#12788=CARTESIAN_POINT('Ctrl Pts',(12.6000000000242,1.90428042250026,0.604702508168697));
#12789=CARTESIAN_POINT('',(12.6,-1.8038302225439,0.7));
#12790=CARTESIAN_POINT('',(12.6,-0.996884774049031,0.7));
#12791=CARTESIAN_POINT('Ctrl Pts',(12.6000000000242,-1.90428042250026,0.604702508168697));
#12792=CARTESIAN_POINT('Ctrl Pts',(12.5999999967566,-1.90390613686288,0.612608546261599));
#12793=CARTESIAN_POINT('Ctrl Pts',(12.6000030637542,-1.90256112855112,0.620429349781532));
#12794=CARTESIAN_POINT('Ctrl Pts',(12.6000044618611,-1.90032851942705,0.628004813168584));
#12795=CARTESIAN_POINT('Ctrl Pts',(12.6000051410147,-1.89924399238468,0.63168472059761));
#12796=CARTESIAN_POINT('Ctrl Pts',(12.6000055125137,-1.89794920179963,0.635306724151721));
#12797=CARTESIAN_POINT('Ctrl Pts',(12.6000054780251,-1.8964494555225,0.638851301608537));
#12798=CARTESIAN_POINT('Ctrl Pts',(12.6000054068101,-1.89335265044601,0.64617044994032));
#12799=CARTESIAN_POINT('Ctrl Pts',(12.6000033360581,-1.88942004582711,0.653077891556402));
#12800=CARTESIAN_POINT('Ctrl Pts',(12.6000021947065,-1.88472046879005,0.659412676045522));
#12801=CARTESIAN_POINT('Ctrl Pts',(12.6000018847951,-1.88344439178375,0.661132761228218));
#12802=CARTESIAN_POINT('Ctrl Pts',(12.6000016718208,-1.88211149822114,0.662810505670431));
#12803=CARTESIAN_POINT('Ctrl Pts',(12.6000016744967,-1.88072259784382,0.664442334323417));
#12804=CARTESIAN_POINT('Ctrl Pts',(12.6000016781594,-1.87882150924004,0.666675936463772));
#12805=CARTESIAN_POINT('Ctrl Pts',(12.6000020841502,-1.87681550570489,0.668823545630641));
#12806=CARTESIAN_POINT('Ctrl Pts',(12.6000026366798,-1.87471194035196,0.670881441794774));
#12807=CARTESIAN_POINT('Ctrl Pts',(12.6000041308351,-1.86902346102148,0.676446422116204));
#12808=CARTESIAN_POINT('Ctrl Pts',(12.600006461375,-1.86269053299793,0.681293522350018));
#12809=CARTESIAN_POINT('Ctrl Pts',(12.6000072160154,-1.85587841208407,0.685370830723365));
#12810=CARTESIAN_POINT('Ctrl Pts',(12.6000077023835,-1.85148797774957,0.687998669380522));
#12811=CARTESIAN_POINT('Ctrl Pts',(12.6000076405209,-1.84689749427555,0.690306084934615));
#12812=CARTESIAN_POINT('Ctrl Pts',(12.6000070464578,-1.84214500723865,0.692269637845719));
#12813=CARTESIAN_POINT('Ctrl Pts',(12.6000061272438,-1.8347913233911,0.69530790964196));
#12814=CARTESIAN_POINT('Ctrl Pts',(12.6000039197963,-1.82713360831075,0.697490862850871));
#12815=CARTESIAN_POINT('Ctrl Pts',(12.6000021173902,-1.81932000848244,0.698749700991972));
#12816=CARTESIAN_POINT('Ctrl Pts',(12.6000009388424,-1.81421089282246,0.699572823470905));
#12817=CARTESIAN_POINT('Ctrl Pts',(12.6,-1.80903450780073,0.7));
#12818=CARTESIAN_POINT('Ctrl Pts',(12.6,-1.80383022254432,0.7));
#12819=CARTESIAN_POINT('Ctrl Pts',(12.4277899437912,-1.91498765980368,8.1061082099175E-6));
#12820=CARTESIAN_POINT('Ctrl Pts',(12.4185093097394,-1.90440735427916,0.201956437811591));
#12821=CARTESIAN_POINT('Ctrl Pts',(12.4092288296506,-1.89382707230216,0.403904777849331));
#12822=CARTESIAN_POINT('Ctrl Pts',(12.3999485057213,-1.88324681432718,0.605853126346544));
#12823=CARTESIAN_POINT('Ctrl Pts',(11.2514531524596,-1.79377193015415,-0.000335869645892519));
#12824=CARTESIAN_POINT('Ctrl Pts',(11.2440495594319,-1.78319067664719,0.201611894978303));
#12825=CARTESIAN_POINT('Ctrl Pts',(11.2366461029568,-1.77260943823668,0.403559665746509));
#12826=CARTESIAN_POINT('Ctrl Pts',(11.2292427771396,-1.76202821861547,0.605507441576721));
#12827=CARTESIAN_POINT('Ctrl Pts',(10.0755218259154,-1.69940246002113,-0.00057195363688788));
#12828=CARTESIAN_POINT('Ctrl Pts',(10.0699958446785,-1.68882059084335,0.201375418496625));
#12829=CARTESIAN_POINT('Ctrl Pts',(10.0644699805481,-1.67823873210945,0.403322794723726));
#12830=CARTESIAN_POINT('Ctrl Pts',(10.0589442279885,-1.66765688783508,0.605270174140068));
#12831=CARTESIAN_POINT('Ctrl Pts',(8.90001330805802,-1.62424530699552,-0.000736768987564917));
#12832=CARTESIAN_POINT('Ctrl Pts',(8.89636559238287,-1.61366301035882,0.201210329036737));
#12833=CARTESIAN_POINT('Ctrl Pts',(8.89271797406169,-1.60308072296431,0.403157429313698));
#12834=CARTESIAN_POINT('Ctrl Pts',(8.88907045450167,-1.59249844499155,0.605104531878289));
#12835=CARTESIAN_POINT('Ctrl Pts',(8.9000000009702,-1.5932011715731,0.605106081469384));
#12836=CARTESIAN_POINT('Ctrl Pts',(10.0684994345535,-1.66840362346204,0.605023135335662));
#12837=CARTESIAN_POINT('Ctrl Pts',(11.2356615742313,-1.76272273105624,0.604904457271936));
#12838=CARTESIAN_POINT('Ctrl Pts',(12.4,-1.8833055216247,0.604732563714112));
#12839=CARTESIAN_POINT('Ctrl Pts',(12.8889963716306,-1.96391015057091,2.25514051876985E-16));
#12840=CARTESIAN_POINT('Ctrl Pts',(12.8789974396847,-1.95334878321431,0.201594505485581));
#12841=CARTESIAN_POINT('Ctrl Pts',(12.8689986695879,-1.94278744208821,0.403189020401051));
#12842=CARTESIAN_POINT('Ctrl Pts',(12.8590000636394,-1.93222612769726,0.604783544887274));
#12843=CARTESIAN_POINT('Ctrl Pts',(12.792662965057,-1.95339909479377,-3.05216148415599E-5));
#12844=CARTESIAN_POINT('Ctrl Pts',(12.7828174539371,-1.94283764251598,0.201563933758495));
#12845=CARTESIAN_POINT('Ctrl Pts',(12.7729721028852,-1.93227621586528,0.403158398317997));
#12846=CARTESIAN_POINT('Ctrl Pts',(12.7631269141758,-1.92171481533493,0.604752872200892));
#12847=CARTESIAN_POINT('Ctrl Pts',(12.6963322449993,-1.94307475200589,-6.02899321993968E-5));
#12848=CARTESIAN_POINT('Ctrl Pts',(12.6866401583647,-1.93251321719056,0.201534116532542));
#12849=CARTESIAN_POINT('Ctrl Pts',(12.6769482300299,-1.92195170741534,0.403128531945268));
#12850=CARTESIAN_POINT('Ctrl Pts',(12.6672564622455,-1.91139022316239,0.604722956439736));
#12851=CARTESIAN_POINT('Ctrl Pts',(12.6000042264769,-1.9329329264796,-8.93242901516475E-5));
#12852=CARTESIAN_POINT('Ctrl Pts',(12.5904655680581,-1.92237131142302,0.201505034443145));
#12853=CARTESIAN_POINT('Ctrl Pts',(12.5809270661843,-1.91180972083551,0.403099401891705));
#12854=CARTESIAN_POINT('Ctrl Pts',(12.5713887230828,-1.90124815518829,0.604693778185974));
#12855=CARTESIAN_POINT('',(12.8572578715866,-1.93204080633595,0.60466226999893));
#12856=CARTESIAN_POINT('Ctrl Pts',(12.6000000000242,-1.90428042250026,0.604702508168697));
#12857=CARTESIAN_POINT('Ctrl Pts',(12.6857696261193,-1.91338852735451,0.604689390578107));
#12858=CARTESIAN_POINT('Ctrl Pts',(12.7715225733429,-1.92264108900731,0.604675979983877));
#12859=CARTESIAN_POINT('Ctrl Pts',(12.8572578715866,-1.93204080633595,0.60466226999893));
#12860=CARTESIAN_POINT('Ctrl Pts',(12.8572578715866,-1.93204080633595,0.604662269998931));
#12861=CARTESIAN_POINT('Ctrl Pts',(12.867837444884,-1.94266422047353,0.403108198925376));
#12862=CARTESIAN_POINT('Ctrl Pts',(12.8784169445746,-1.95328733374019,0.201554108835025));
#12863=CARTESIAN_POINT('Ctrl Pts',(12.8889963716306,-1.96391015057091,-1.13624387676481E-16));
#12864=CARTESIAN_POINT('Ctrl Pts',(12.4102890066107,-1.7839488953552,0.7));
#12865=CARTESIAN_POINT('Ctrl Pts',(11.2423261062923,-1.6629989551888,0.7));
#12866=CARTESIAN_POINT('Ctrl Pts',(10.0717272052363,-1.56846077660453,0.7));
#12867=CARTESIAN_POINT('Ctrl Pts',(8.89999999999993,-1.49312521822106,0.7));
#12868=CARTESIAN_POINT('Ctrl Pts',(12.4072999778185,-1.81281269415102,0.7));
#12869=CARTESIAN_POINT('Ctrl Pts',(11.2397765858669,-1.69187462084457,0.699998757165067));
#12870=CARTESIAN_POINT('Ctrl Pts',(10.0695527221263,-1.59734372851255,0.700000594792869));
#12871=CARTESIAN_POINT('Ctrl Pts',(8.89814271406455,-1.52201240649035,0.7));
#12872=CARTESIAN_POINT('Ctrl Pts',(12.4021203845267,-1.86282985658401,0.676448561733929));
#12873=CARTESIAN_POINT('Ctrl Pts',(11.2353531757414,-1.74191593276004,0.676505236381959));
#12874=CARTESIAN_POINT('Ctrl Pts',(10.0657879841113,-1.64739716848489,0.676543604639643));
#12875=CARTESIAN_POINT('Ctrl Pts',(8.89492397206972,-1.57207492202614,0.676570833338327));
#12876=CARTESIAN_POINT('Ctrl Pts',(12.400106093269,-1.88228102337346,0.626471792264191));
#12877=CARTESIAN_POINT('Ctrl Pts',(11.2336287644773,-1.76143987438699,0.626617923584012));
#12878=CARTESIAN_POINT('Ctrl Pts',(10.0643137348541,-1.66697079985262,0.626717999675944));
#12879=CARTESIAN_POINT('Ctrl Pts',(8.89366330605793,-1.59168261717615,0.626788336025017));
#12880=CARTESIAN_POINT('Ctrl Pts',(12.4,-1.8833055216247,0.604732563714112));
#12881=CARTESIAN_POINT('Ctrl Pts',(11.2335332423564,-1.7625023138725,0.604904771481731));
#12882=CARTESIAN_POINT('Ctrl Pts',(10.0642324382527,-1.66805889332185,0.605023569028795));
#12883=CARTESIAN_POINT('Ctrl Pts',(8.89359217382714,-1.59278896817116,0.605106535971077));
#12884=CARTESIAN_POINT('Ctrl Pts',(12.400000003046,-1.78288409409898,0.7));
#12885=CARTESIAN_POINT('Ctrl Pts',(11.235451325406,-1.66244391065713,0.7));
#12886=CARTESIAN_POINT('Ctrl Pts',(10.0682865064676,-1.56823955876321,0.7));
#12887=CARTESIAN_POINT('Ctrl Pts',(8.89999999999993,-1.49312521822106,0.7));
#12888=CARTESIAN_POINT('Ctrl Pts',(12.8681436286308,-1.83274446434879,0.7));
#12889=CARTESIAN_POINT('Ctrl Pts',(12.7787800350189,-1.82294762441299,0.7));
#12890=CARTESIAN_POINT('Ctrl Pts',(12.6893984576578,-1.8133105623702,0.7));
#12891=CARTESIAN_POINT('Ctrl Pts',(12.6,-1.80383022254431,0.7));
#12892=CARTESIAN_POINT('Ctrl Pts',(12.8649798835675,-1.86160311979107,0.7));
#12893=CARTESIAN_POINT('Ctrl Pts',(12.7756511334299,-1.85180730951691,0.699999896874207));
#12894=CARTESIAN_POINT('Ctrl Pts',(12.686303642571,-1.84217134991284,0.700000098415946));
#12895=CARTESIAN_POINT('Ctrl Pts',(12.5969393303221,-1.83269196733649,0.7));
#12896=CARTESIAN_POINT('Ctrl Pts',(12.8594976525144,-1.91161025179704,0.676425356750174));
#12897=CARTESIAN_POINT('Ctrl Pts',(12.7702288461641,-1.90181652272411,0.676430055978541));
#12898=CARTESIAN_POINT('Ctrl Pts',(12.6809412203008,-1.89218243450198,0.676434576658958));
#12899=CARTESIAN_POINT('Ctrl Pts',(12.5916356538948,-1.88270499442535,0.67643906321291));
#12900=CARTESIAN_POINT('Ctrl Pts',(12.8573684983393,-1.93103170500986,0.626412260100396));
#12901=CARTESIAN_POINT('Ctrl Pts',(12.7681225846323,-1.92124403769089,0.626424372515079));
#12902=CARTESIAN_POINT('Ctrl Pts',(12.6788572782757,-1.91161594713487,0.626436135819418));
#12903=CARTESIAN_POINT('Ctrl Pts',(12.5895741974899,-1.90214427893475,0.626447702441804));
#12904=CARTESIAN_POINT('Ctrl Pts',(12.8572578715866,-1.93204080633595,0.60466226999893));
#12905=CARTESIAN_POINT('Ctrl Pts',(12.7680127446979,-1.92225628370762,0.604676541242762));
#12906=CARTESIAN_POINT('Ctrl Pts',(12.6787484942245,-1.91263121188365,0.60469048808123));
#12907=CARTESIAN_POINT('Ctrl Pts',(12.5894662143615,-1.9031625467727,0.604704117718382));
#12908=CARTESIAN_POINT('',(12.8681436286308,-1.83274446434879,0.7));
#12909=CARTESIAN_POINT('Ctrl Pts',(12.8681436286308,-1.83274446434879,0.7));
#12910=CARTESIAN_POINT('Ctrl Pts',(12.7787800350189,-1.82294762441299,0.7));
#12911=CARTESIAN_POINT('Ctrl Pts',(12.6893984576578,-1.8133105623702,0.7));
#12912=CARTESIAN_POINT('Ctrl Pts',(12.6,-1.80383022254431,0.7));
#12913=CARTESIAN_POINT('Origin',(12.8681436286308,-1.83274446434879,0.6));
#12914=CARTESIAN_POINT('Origin',(6.87409734069396,-2.22251806091942E-16,
0.7));
#12915=CARTESIAN_POINT('Ctrl Pts',(8.9,1.49312521822106,0.7));
#12916=CARTESIAN_POINT('Ctrl Pts',(10.0682865064677,1.56823955876321,0.7));
#12917=CARTESIAN_POINT('Ctrl Pts',(11.2354513254061,1.66244391065714,0.7));
#12918=CARTESIAN_POINT('Ctrl Pts',(12.4000000030461,1.78288409409899,0.7));
#12919=CARTESIAN_POINT('Origin',(6.87409734069396,-2.22251806091942E-16,
0.7));
#12920=CARTESIAN_POINT('',(12.8681436286308,1.83274446434879,0.7));
#12921=CARTESIAN_POINT('Ctrl Pts',(12.6,1.80383022254432,0.7));
#12922=CARTESIAN_POINT('Ctrl Pts',(12.6893984576578,1.8133105623702,0.7));
#12923=CARTESIAN_POINT('Ctrl Pts',(12.7787800350189,1.82294762441299,0.7));
#12924=CARTESIAN_POINT('Ctrl Pts',(12.8681436286308,1.83274446434879,0.7));
#12925=CARTESIAN_POINT('',(12.8681436286308,1.1,0.7));
#12926=CARTESIAN_POINT('Ctrl Pts',(8.9,1.49312521822106,0.7));
#12927=CARTESIAN_POINT('Ctrl Pts',(10.0717272052363,1.56846077660453,0.7));
#12928=CARTESIAN_POINT('Ctrl Pts',(11.2423261062923,1.6629989551888,0.7));
#12929=CARTESIAN_POINT('Ctrl Pts',(12.4102890066107,1.7839488953552,0.7));
#12930=CARTESIAN_POINT('Ctrl Pts',(8.89814271406461,1.52201240649035,0.7));
#12931=CARTESIAN_POINT('Ctrl Pts',(10.0695527221263,1.59734372851256,0.700000594792869));
#12932=CARTESIAN_POINT('Ctrl Pts',(11.2397765858669,1.69187462084457,0.699998757165067));
#12933=CARTESIAN_POINT('Ctrl Pts',(12.4072999778185,1.81281269415102,0.7));
#12934=CARTESIAN_POINT('Ctrl Pts',(8.89492397206979,1.57207492202615,0.676570833338327));
#12935=CARTESIAN_POINT('Ctrl Pts',(10.0657879841114,1.64739716848489,0.676543604639644));
#12936=CARTESIAN_POINT('Ctrl Pts',(11.2353531757414,1.74191593276004,0.676505236381959));
#12937=CARTESIAN_POINT('Ctrl Pts',(12.4021203845267,1.86282985658401,0.676448561733929));
#12938=CARTESIAN_POINT('Ctrl Pts',(8.89366330605799,1.59168261717616,0.626788336025017));
#12939=CARTESIAN_POINT('Ctrl Pts',(10.0643137348542,1.66697079985262,0.626717999675944));
#12940=CARTESIAN_POINT('Ctrl Pts',(11.2336287644773,1.761439874387,0.626617923584012));
#12941=CARTESIAN_POINT('Ctrl Pts',(12.400106093269,1.88228102337346,0.626471792264191));
#12942=CARTESIAN_POINT('Ctrl Pts',(8.89359217382721,1.59278896817116,0.605106535971077));
#12943=CARTESIAN_POINT('Ctrl Pts',(10.0642324382527,1.66805889332185,0.605023569028795));
#12944=CARTESIAN_POINT('Ctrl Pts',(11.2335332423565,1.7625023138725,0.604904771481731));
#12945=CARTESIAN_POINT('Ctrl Pts',(12.4,1.8833055216247,0.604732563714112));
#12946=CARTESIAN_POINT('Ctrl Pts',(12.4,1.8833055216247,0.604732563714112));
#12947=CARTESIAN_POINT('Ctrl Pts',(11.2356615742313,1.76272273105624,0.604904457271936));
#12948=CARTESIAN_POINT('Ctrl Pts',(10.0684994345535,1.66840362346204,0.605023135335662));
#12949=CARTESIAN_POINT('Ctrl Pts',(8.90000000097019,1.5932011715731,0.605106081469384));
#12950=CARTESIAN_POINT('Ctrl Pts',(8.90001330805765,1.62424530699444,-0.000736768966955875));
#12951=CARTESIAN_POINT('Ctrl Pts',(8.89636559238262,1.6136630103581,0.201210329050476));
#12952=CARTESIAN_POINT('Ctrl Pts',(8.89271797406156,1.60308072296395,0.403157429320568));
#12953=CARTESIAN_POINT('Ctrl Pts',(8.88907045450167,1.59249844499155,0.605104531878289));
#12954=CARTESIAN_POINT('Ctrl Pts',(10.0755218259151,1.69940246002007,-0.000571953616278766));
#12955=CARTESIAN_POINT('Ctrl Pts',(10.0699958446785,1.68882059084265,0.201375418510364));
#12956=CARTESIAN_POINT('Ctrl Pts',(10.0644699805483,1.67823873210911,0.403322794730596));
#12957=CARTESIAN_POINT('Ctrl Pts',(10.0589442279888,1.6676568878351,0.605270174140069));
#12958=CARTESIAN_POINT('Ctrl Pts',(11.2514531524595,1.79377193015312,-0.000335869625283423));
#12959=CARTESIAN_POINT('Ctrl Pts',(11.244049559432,1.78319067664652,0.201611894992042));
#12960=CARTESIAN_POINT('Ctrl Pts',(11.2366461029572,1.77260943823637,0.403559665753379));
#12961=CARTESIAN_POINT('Ctrl Pts',(11.2292427771402,1.76202821861552,0.605507441576721));
#12962=CARTESIAN_POINT('Ctrl Pts',(12.4277899437912,1.9149876598027,8.10612881915578E-6));
#12963=CARTESIAN_POINT('Ctrl Pts',(12.4185093097397,1.90440735427854,0.201956437825331));
#12964=CARTESIAN_POINT('Ctrl Pts',(12.4092288296513,1.89382707230189,0.403904777856201));
#12965=CARTESIAN_POINT('Ctrl Pts',(12.3999485057223,1.88324681432728,0.605853126346545));
#12966=CARTESIAN_POINT('Ctrl Pts',(12.6000042264759,1.9329329264795,-8.93242901520291E-5));
#12967=CARTESIAN_POINT('Ctrl Pts',(12.5904655680574,1.92237131142328,0.201505034436202));
#12968=CARTESIAN_POINT('Ctrl Pts',(12.580927066184,1.91180972083614,0.403099401877819));
#12969=CARTESIAN_POINT('Ctrl Pts',(12.5713887230828,1.90124815518927,0.604693778165146));
#12970=CARTESIAN_POINT('Ctrl Pts',(12.6963322449987,1.94307475200582,-6.02899321996874E-5));
#12971=CARTESIAN_POINT('Ctrl Pts',(12.6866401583644,1.93251321719085,0.201534116525599));
#12972=CARTESIAN_POINT('Ctrl Pts',(12.6769482300299,1.921951707416,0.403128531931383));
#12973=CARTESIAN_POINT('Ctrl Pts',(12.6672564622458,1.91139022316341,0.604722956418908));
#12974=CARTESIAN_POINT('Ctrl Pts',(12.7926629650567,1.95339909479374,-3.05216148420481E-5));
#12975=CARTESIAN_POINT('Ctrl Pts',(12.7828174539371,1.94283764251631,0.201563933751552));
#12976=CARTESIAN_POINT('Ctrl Pts',(12.7729721028855,1.93227621586597,0.403158398304112));
#12977=CARTESIAN_POINT('Ctrl Pts',(12.7631269141765,1.92171481533599,0.604752872180064));
#12978=CARTESIAN_POINT('Ctrl Pts',(12.8889963716306,1.96391015057091,-1.66533453693773E-16));
#12979=CARTESIAN_POINT('Ctrl Pts',(12.878997439685,1.95334878321468,0.201594505478638));
#12980=CARTESIAN_POINT('Ctrl Pts',(12.8689986695886,1.94278744208894,0.403189020387166));
#12981=CARTESIAN_POINT('Ctrl Pts',(12.8590000636404,1.93222612769835,0.604783544866446));
#12982=CARTESIAN_POINT('',(12.8572578715866,1.93204080633595,0.60466226999893));
#12983=CARTESIAN_POINT('Ctrl Pts',(12.8889963716306,1.96391015057091,-3.88144377749811E-17));
#12984=CARTESIAN_POINT('Ctrl Pts',(12.8784169445746,1.95328733374019,0.201554108835021));
#12985=CARTESIAN_POINT('Ctrl Pts',(12.867837444884,1.94266422047353,0.403108198925375));
#12986=CARTESIAN_POINT('Ctrl Pts',(12.8572578715866,1.93204080633595,0.604662269998929));
#12987=CARTESIAN_POINT('Ctrl Pts',(12.8572578715866,1.93204080633595,0.60466226999893));
#12988=CARTESIAN_POINT('Ctrl Pts',(12.7715225733429,1.92264108900731,0.604675979983877));
#12989=CARTESIAN_POINT('Ctrl Pts',(12.6857696261193,1.91338852735451,0.604689390578107));
#12990=CARTESIAN_POINT('Ctrl Pts',(12.6000000000242,1.90428042250026,0.604702508168697));
#12991=CARTESIAN_POINT('Origin',(8.7,1.68851851851852,0.));
#12992=CARTESIAN_POINT('',(8.7,-1.5805153611151,0.605119933308333));
#12993=CARTESIAN_POINT('Ctrl Pts',(8.7,-1.5805153611151,0.605119933308333));
#12994=CARTESIAN_POINT('Ctrl Pts',(8.7,-1.58569938832865,0.504197823486131));
#12995=CARTESIAN_POINT('Ctrl Pts',(8.7,-1.59088373519313,0.403275164205241));
#12996=CARTESIAN_POINT('Ctrl Pts',(8.7,-1.60124586355191,0.201568897935389));
#12997=CARTESIAN_POINT('Ctrl Pts',(8.7,-1.60642370224807,0.10078416210737));
#12998=CARTESIAN_POINT('Ctrl Pts',(8.7,-1.61160179736194,0.));
#12999=CARTESIAN_POINT('',(8.7,-1.48045180431786,0.7));
#13000=CARTESIAN_POINT('Ctrl Pts',(8.70000000036779,-1.48045180452391,0.7));
#13001=CARTESIAN_POINT('Ctrl Pts',(8.70000000202598,-1.48836706478042,0.699999999180279));
#13002=CARTESIAN_POINT('Ctrl Pts',(8.70000127066624,-1.49622113223642,0.699007614827928));
#13003=CARTESIAN_POINT('Ctrl Pts',(8.70000237141531,-1.50387364922569,0.697121884028934));
#13004=CARTESIAN_POINT('Ctrl Pts',(8.70000291188189,-1.50763102664002,0.696195992283305));
#13005=CARTESIAN_POINT('Ctrl Pts',(8.70000341240591,-1.51133980954515,0.695053883793301));
#13006=CARTESIAN_POINT('Ctrl Pts',(8.70000377175886,-1.51498230649063,0.693702880475192));
#13007=CARTESIAN_POINT('Ctrl Pts',(8.70000450976793,-1.52246296255016,0.690928302676144));
#13008=CARTESIAN_POINT('Ctrl Pts',(8.70000452394134,-1.52958344744078,0.687306123577328));
#13009=CARTESIAN_POINT('Ctrl Pts',(8.70000379461986,-1.53619834892264,0.682919715776694));
#13010=CARTESIAN_POINT('Ctrl Pts',(8.70000333219987,-1.54039247012311,0.680138551763745));
#13011=CARTESIAN_POINT('Ctrl Pts',(8.70000258238552,-1.54438316197938,0.67704909562189));
#13012=CARTESIAN_POINT('Ctrl Pts',(8.70000192913237,-1.54812716280968,0.67366362845569));
#13013=CARTESIAN_POINT('Ctrl Pts',(8.70000138361353,-1.55125370412533,0.670836491537814));
#13014=CARTESIAN_POINT('Ctrl Pts',(8.70000090341281,-1.55418891097064,0.66782012731024));
#13015=CARTESIAN_POINT('Ctrl Pts',(8.7000009033621,-1.55691103280728,0.664625500020687));
#13016=CARTESIAN_POINT('Ctrl Pts',(8.7000009032669,-1.56202159382457,0.658627848677152));
#13017=CARTESIAN_POINT('Ctrl Pts',(8.70000241148087,-1.56638404855443,0.652003279246098));
#13018=CARTESIAN_POINT('Ctrl Pts',(8.70000292788623,-1.5699383402149,0.64491699469699));
#13019=CARTESIAN_POINT('Ctrl Pts',(8.70000298354275,-1.57032141040405,0.644153257609021));
#13020=CARTESIAN_POINT('Ctrl Pts',(8.70000303046442,-1.57069504840788,0.643384135640712));
#13021=CARTESIAN_POINT('Ctrl Pts',(8.70000306761332,-1.57105914547653,0.642609822781892));
#13022=CARTESIAN_POINT('Ctrl Pts',(8.70000341208914,-1.57443535963509,0.635429742901602));
#13023=CARTESIAN_POINT('Ctrl Pts',(8.70000263566904,-1.57695592401075,0.627888404173009));
#13024=CARTESIAN_POINT('Ctrl Pts',(8.70000151703179,-1.57856725066757,0.620153930269154));
#13025=CARTESIAN_POINT('Ctrl Pts',(8.70000080174396,-1.57959757782623,0.615208292159515));
#13026=CARTESIAN_POINT('Ctrl Pts',(8.7,-1.58025528705454,0.610183028431161));
#13027=CARTESIAN_POINT('Ctrl Pts',(8.7,-1.5805153611151,0.605119933308333));
#13028=CARTESIAN_POINT('',(8.7,1.48045180431904,0.7));
#13029=CARTESIAN_POINT('',(8.7,0.844259259259259,0.7));
#13030=CARTESIAN_POINT('',(8.7,1.5805153611151,0.605119933308333));
#13031=CARTESIAN_POINT('Ctrl Pts',(8.7,1.5805153611151,0.605119933308333));
#13032=CARTESIAN_POINT('Ctrl Pts',(8.7,1.58010890623597,0.61303275518587));
#13033=CARTESIAN_POINT('Ctrl Pts',(8.70000179355525,1.57873376841273,0.620855553142259));
#13034=CARTESIAN_POINT('Ctrl Pts',(8.7000025961206,1.5764741717406,0.62842799710221));
#13035=CARTESIAN_POINT('Ctrl Pts',(8.70000304562639,1.57520860278123,0.632669218617747));
#13036=CARTESIAN_POINT('Ctrl Pts',(8.70000324668712,1.57366457852079,0.636831947144834));
#13037=CARTESIAN_POINT('Ctrl Pts',(8.70000313318341,1.57185009366145,0.640886032861668));
#13038=CARTESIAN_POINT('Ctrl Pts',(8.70000293045856,1.56860930815545,0.648126888117959));
#13039=CARTESIAN_POINT('Ctrl Pts',(8.70000158438082,1.56454425420738,0.654942317779106));
#13040=CARTESIAN_POINT('Ctrl Pts',(8.70000106269264,1.55971945710293,0.661169479919421));
#13041=CARTESIAN_POINT('Ctrl Pts',(8.70000096439252,1.55881033523018,0.662342845179011));
#13042=CARTESIAN_POINT('Ctrl Pts',(8.70000090351839,1.55787410801649,0.663495254390581));
#13043=CARTESIAN_POINT('Ctrl Pts',(8.70000090409683,1.55691103285321,0.664625500020665));
#13044=CARTESIAN_POINT('Ctrl Pts',(8.70000090523835,1.55501044337284,0.666855993586132));
#13045=CARTESIAN_POINT('Ctrl Pts',(8.70000114361209,1.55300532702719,0.669000219206223));
#13046=CARTESIAN_POINT('Ctrl Pts',(8.70000146777886,1.55090303951829,0.671054438207787));
#13047=CARTESIAN_POINT('Ctrl Pts',(8.70000234447876,1.54521746205001,0.676610015749294));
#13048=CARTESIAN_POINT('Ctrl Pts',(8.70000370702799,1.53888821826629,0.681447385411957));
#13049=CARTESIAN_POINT('Ctrl Pts',(8.70000415375638,1.53207947242364,0.685512859850771));
#13050=CARTESIAN_POINT('Ctrl Pts',(8.70000443876751,1.52773551673798,0.688106618115728));
#13051=CARTESIAN_POINT('Ctrl Pts',(8.70000441165582,1.52319541573235,0.690385508075002));
#13052=CARTESIAN_POINT('Ctrl Pts',(8.70000407315693,1.51849599021366,0.692326230693156));
#13053=CARTESIAN_POINT('Ctrl Pts',(8.70000354533424,1.51116815716702,0.695352407250086));
#13054=CARTESIAN_POINT('Ctrl Pts',(8.70000225790696,1.50353761203248,0.697524030080351));
#13055=CARTESIAN_POINT('Ctrl Pts',(8.70000121423997,1.49575164755759,0.698771658000832));
#13056=CARTESIAN_POINT('Ctrl Pts',(8.70000053774506,1.49070486028667,0.699580358416591));
#13057=CARTESIAN_POINT('Ctrl Pts',(8.70000000144466,1.48559217323052,0.699999999467653));
#13058=CARTESIAN_POINT('Ctrl Pts',(8.70000000036779,1.48045180452391,0.7));
#13059=CARTESIAN_POINT('Ctrl Pts',(8.7,1.61160179736194,0.));
#13060=CARTESIAN_POINT('Ctrl Pts',(8.7,1.60642368739695,0.100784451162898));
#13061=CARTESIAN_POINT('Ctrl Pts',(8.7,1.60124583384883,0.201569476094892));
#13062=CARTESIAN_POINT('Ctrl Pts',(8.7,1.59088370548997,0.403275742430776));
#13063=CARTESIAN_POINT('Ctrl Pts',(8.7,1.58569937347746,0.504198112607714));
#13064=CARTESIAN_POINT('Ctrl Pts',(8.7,1.5805153611151,0.605119933308333));
#13065=CARTESIAN_POINT('Ctrl Pts',(8.7100201910492,-1.61222456240079,1.33887903992595E-6));
#13066=CARTESIAN_POINT('Ctrl Pts',(8.70667727354472,-1.60164608969543,0.201874135619687));
#13067=CARTESIAN_POINT('Ctrl Pts',(8.70333445073708,-1.59106762573893,0.40374693439627));
#13068=CARTESIAN_POINT('Ctrl Pts',(8.69999172399519,-1.58048917070122,0.605619735240497));
#13069=CARTESIAN_POINT('Ctrl Pts',(7.30266630830786,-1.52469223633113,-0.000186944012493601));
#13070=CARTESIAN_POINT('Ctrl Pts',(7.3015714609838,-1.51411327886182,0.201685539385837));
#13071=CARTESIAN_POINT('Ctrl Pts',(7.30047669312962,-1.50353432123569,0.403558023359813));
#13072=CARTESIAN_POINT('Ctrl Pts',(7.2993819983171,-1.49295537435081,0.605430507723141));
#13073=CARTESIAN_POINT('Ctrl Pts',(5.89591889571946,-1.46411055243784,-0.000276130330627546));
#13074=CARTESIAN_POINT('Ctrl Pts',(5.8970730573458,-1.45353136553189,0.201596203763285));
#13075=CARTESIAN_POINT('Ctrl Pts',(5.89822728315403,-1.44295217665945,0.403468537584815));
#13076=CARTESIAN_POINT('Ctrl Pts',(5.89938156763751,-1.43237299696387,0.60534087113472));
#13077=CARTESIAN_POINT('Ctrl Pts',(4.48978738186403,-1.41740792524342,-0.000330195618103912));
#13078=CARTESIAN_POINT('Ctrl Pts',(4.49319153668887,-1.4068286019831,0.201542048187911));
#13079=CARTESIAN_POINT('Ctrl Pts',(4.49659574248722,-1.39624928130228,0.403414291272231));
#13080=CARTESIAN_POINT('Ctrl Pts',(4.5,-1.3856699632509,0.605286533625018));
#13081=CARTESIAN_POINT('Ctrl Pts',(4.50000000014037,-1.38566996330298,0.605286533623957));
#13082=CARTESIAN_POINT('Ctrl Pts',(5.90109530155974,-1.43243455365708,0.605259331490037));
#13083=CARTESIAN_POINT('Ctrl Pts',(7.30150776148394,-1.49309969195427,0.605214402664297));
#13084=CARTESIAN_POINT('Ctrl Pts',(8.7,-1.5805153611151,0.605119933308333));
#13085=CARTESIAN_POINT('Ctrl Pts',(8.7062300060629,-1.48084102486261,0.7));
#13086=CARTESIAN_POINT('Ctrl Pts',(7.30535837857749,-1.39328148786737,0.7));
#13087=CARTESIAN_POINT('Ctrl Pts',(5.90286553803659,-1.3325543763676,0.7));
#13088=CARTESIAN_POINT('Ctrl Pts',(4.5,-1.28575421950843,0.7));
#13089=CARTESIAN_POINT('Ctrl Pts',(8.7044244076592,-1.50972892972339,0.7));
#13090=CARTESIAN_POINT('Ctrl Pts',(7.30392377861185,-1.42217417124324,0.699999322371676));
#13091=CARTESIAN_POINT('Ctrl Pts',(5.90170976758769,-1.36144968116949,0.700000194339816));
#13092=CARTESIAN_POINT('Ctrl Pts',(4.49903600403804,-1.314650633636,0.7));
#13093=CARTESIAN_POINT('Ctrl Pts',(8.70129509098077,-1.55979510296572,0.676577193851887));
#13094=CARTESIAN_POINT('Ctrl Pts',(7.30143307762773,-1.47225060169427,0.676608218952397));
#13095=CARTESIAN_POINT('Ctrl Pts',(5.89970879741633,-1.41153023905743,0.676622651488038));
#13096=CARTESIAN_POINT('Ctrl Pts',(4.49736521340071,-1.36473368385825,0.676631564755462));
#13097=CARTESIAN_POINT('Ctrl Pts',(8.70006933407556,-1.57940608001781,0.626799670546273));
#13098=CARTESIAN_POINT('Ctrl Pts',(7.3004573192207,-1.49190036240803,0.626879818917698));
#13099=CARTESIAN_POINT('Ctrl Pts',(5.89892183391985,-1.43119871194172,0.62691759730524));
#13100=CARTESIAN_POINT('Ctrl Pts',(4.49670869913724,-1.38441313147668,0.626940642142451));
#13101=CARTESIAN_POINT('Ctrl Pts',(8.7,-1.5805153611151,0.605119933308333));
#13102=CARTESIAN_POINT('Ctrl Pts',(7.30039998287682,-1.49303044794594,0.605214477495697));
#13103=CARTESIAN_POINT('Ctrl Pts',(5.89887670103551,-1.4323384618751,0.605259402637312));
#13104=CARTESIAN_POINT('Ctrl Pts',(4.49667047719213,-1.38555885946567,0.605286598232956));
#13105=CARTESIAN_POINT('Ctrl Pts',(8.70000000036771,-1.48045180452391,0.7));
#13106=CARTESIAN_POINT('Ctrl Pts',(7.30120024114866,-1.39310147361351,0.7));
#13107=CARTESIAN_POINT('Ctrl Pts',(5.90078591724148,-1.332484999384,0.7));
#13108=CARTESIAN_POINT('Ctrl Pts',(4.5,-1.28575421950843,0.7));
#13109=CARTESIAN_POINT('Origin',(6.87409734069396,-2.22251806091942E-16,
0.7));
#13110=CARTESIAN_POINT('Ctrl Pts',(4.5,1.28575421950843,0.7));
#13111=CARTESIAN_POINT('Ctrl Pts',(5.9007859172415,1.332484999384,0.7));
#13112=CARTESIAN_POINT('Ctrl Pts',(7.30120024114871,1.39310147361351,0.7));
#13113=CARTESIAN_POINT('Ctrl Pts',(8.70000000036779,1.48045180452391,0.7));
#13114=CARTESIAN_POINT('Ctrl Pts',(4.5,1.28575421950843,0.7));
#13115=CARTESIAN_POINT('Ctrl Pts',(5.90286553803659,1.3325543763676,0.7));
#13116=CARTESIAN_POINT('Ctrl Pts',(7.30535837857749,1.39328148786737,0.7));
#13117=CARTESIAN_POINT('Ctrl Pts',(8.7062300060629,1.48084102486261,0.7));
#13118=CARTESIAN_POINT('Ctrl Pts',(4.49903600403804,1.314650633636,0.7));
#13119=CARTESIAN_POINT('Ctrl Pts',(5.90170976758769,1.36144968116949,0.700000194339816));
#13120=CARTESIAN_POINT('Ctrl Pts',(7.30392377861185,1.42217417124324,0.699999322371676));
#13121=CARTESIAN_POINT('Ctrl Pts',(8.7044244076592,1.50972892972339,0.7));
#13122=CARTESIAN_POINT('Ctrl Pts',(4.49736521340071,1.36473368385825,0.676631564755462));
#13123=CARTESIAN_POINT('Ctrl Pts',(5.89970879741633,1.41153023905743,0.676622651488038));
#13124=CARTESIAN_POINT('Ctrl Pts',(7.30143307762774,1.47225060169427,0.676608218952397));
#13125=CARTESIAN_POINT('Ctrl Pts',(8.70129509098078,1.55979510296572,0.676577193851887));
#13126=CARTESIAN_POINT('Ctrl Pts',(4.49670869913724,1.38441313147668,0.626940642142451));
#13127=CARTESIAN_POINT('Ctrl Pts',(5.89892183391985,1.43119871194172,0.626917597305239));
#13128=CARTESIAN_POINT('Ctrl Pts',(7.3004573192207,1.49190036240803,0.626879818917698));
#13129=CARTESIAN_POINT('Ctrl Pts',(8.70006933407556,1.57940608001781,0.626799670546273));
#13130=CARTESIAN_POINT('Ctrl Pts',(4.49667047719213,1.38555885946567,0.605286598232956));
#13131=CARTESIAN_POINT('Ctrl Pts',(5.89887670103551,1.4323384618751,0.605259402637312));
#13132=CARTESIAN_POINT('Ctrl Pts',(7.30039998287682,1.49303044794594,0.605214477495697));
#13133=CARTESIAN_POINT('Ctrl Pts',(8.7,1.5805153611151,0.605119933308333));
#13134=CARTESIAN_POINT('Ctrl Pts',(8.7,1.5805153611151,0.605119933308333));
#13135=CARTESIAN_POINT('Ctrl Pts',(7.30150776148394,1.49309969195427,0.605214402664297));
#13136=CARTESIAN_POINT('Ctrl Pts',(5.90109530155974,1.43243455365708,0.605259331490037));
#13137=CARTESIAN_POINT('Ctrl Pts',(4.50000000014037,1.38566996330298,0.605286533623957));
#13138=CARTESIAN_POINT('Ctrl Pts',(4.48978738186405,1.41740792524342,-0.00033019561810394));
#13139=CARTESIAN_POINT('Ctrl Pts',(4.49319153668889,1.40682860198312,0.201542048187577));
#13140=CARTESIAN_POINT('Ctrl Pts',(4.49659574248723,1.39624928130232,0.403414291271564));
#13141=CARTESIAN_POINT('Ctrl Pts',(4.5,1.38566996325095,0.605286533624017));
#13142=CARTESIAN_POINT('Ctrl Pts',(5.89591889571947,1.46411055243784,-0.000276130330627574));
#13143=CARTESIAN_POINT('Ctrl Pts',(5.89707305734581,1.45353136553191,0.201596203762952));
#13144=CARTESIAN_POINT('Ctrl Pts',(5.89822728315404,1.44295217665948,0.403468537584147));
#13145=CARTESIAN_POINT('Ctrl Pts',(5.89938156763751,1.43237299696393,0.605340871133719));
#13146=CARTESIAN_POINT('Ctrl Pts',(7.30266630830786,1.52469223633113,-0.000186944012493549));
#13147=CARTESIAN_POINT('Ctrl Pts',(7.3015714609838,1.51411327886184,0.201685539385503));
#13148=CARTESIAN_POINT('Ctrl Pts',(7.30047669312963,1.50353432123572,0.403558023359145));
#13149=CARTESIAN_POINT('Ctrl Pts',(7.29938199831711,1.49295537435086,0.60543050772214));
#13150=CARTESIAN_POINT('Ctrl Pts',(8.7100201910492,1.61222456240079,1.33887903989646E-6));
#13151=CARTESIAN_POINT('Ctrl Pts',(8.70667727354472,1.60164608969545,0.201874135619353));
#13152=CARTESIAN_POINT('Ctrl Pts',(8.7033344507371,1.59106762573896,0.403746934395602));
#13153=CARTESIAN_POINT('Ctrl Pts',(8.6999917239952,1.58048917070127,0.605619735239495));
#13154=CARTESIAN_POINT('Origin',(4.3,1.48481481481482,0.));
#13155=CARTESIAN_POINT('',(4.3,-1.37908752581626,0.605290299758539));
#13156=CARTESIAN_POINT('Ctrl Pts',(4.3,-1.37908752581626,0.605290299758539));
#13157=CARTESIAN_POINT('Ctrl Pts',(4.3,-1.38444464017247,0.504222347694443));
#13158=CARTESIAN_POINT('Ctrl Pts',(4.3,-1.38980163214303,0.403154389143214));
#13159=CARTESIAN_POINT('Ctrl Pts',(4.3,-1.40049562949383,0.201390955816302));
#13160=CARTESIAN_POINT('Ctrl Pts',(4.3,-1.40583263576898,0.100695481088992));
#13161=CARTESIAN_POINT('Ctrl Pts',(4.3,-1.41116952203211,0.));
#13162=CARTESIAN_POINT('Ctrl Pts',(4.30000000005992,-1.27917501058303,0.7));
#13163=CARTESIAN_POINT('Ctrl Pts',(4.30000000048661,-1.28708628524264,0.699999999884766));
#13164=CARTESIAN_POINT('Ctrl Pts',(4.30000064978116,-1.29493415608545,0.69900616264686));
#13165=CARTESIAN_POINT('Ctrl Pts',(4.30000121018478,-1.30257825621016,0.697119208693397));
#13166=CARTESIAN_POINT('Ctrl Pts',(4.30000152558655,-1.30688044586137,0.696057208766858));
#13167=CARTESIAN_POINT('Ctrl Pts',(4.30000181105247,-1.31111814675806,0.694711271736901));
#13168=CARTESIAN_POINT('Ctrl Pts',(4.30000199036827,-1.31526464671957,0.693092387263961));
#13169=CARTESIAN_POINT('Ctrl Pts',(4.30000231141323,-1.32268849323592,0.690193954859197));
#13170=CARTESIAN_POINT('Ctrl Pts',(4.30000222777046,-1.32973966400828,0.686455190804221));
#13171=CARTESIAN_POINT('Ctrl Pts',(4.30000179417102,-1.33627196700415,0.681957645816867));
#13172=CARTESIAN_POINT('Ctrl Pts',(4.30000155535849,-1.33986974800182,0.679480543652151));
#13173=CARTESIAN_POINT('Ctrl Pts',(4.30000121902461,-1.34330986828215,0.67677238407294));
#13174=CARTESIAN_POINT('Ctrl Pts',(4.30000092191081,-1.34656397897095,0.673841242448196));
#13175=CARTESIAN_POINT('Ctrl Pts',(4.30000063243573,-1.34973442737118,0.670985459666446));
#13176=CARTESIAN_POINT('Ctrl Pts',(4.30000037658882,-1.35270906921767,0.667935271966333));
#13177=CARTESIAN_POINT('Ctrl Pts',(4.30000037869864,-1.35546536049262,0.66470214425512));
#13178=CARTESIAN_POINT('Ctrl Pts',(4.30000038260995,-1.36057515211559,0.658708362304413));
#13179=CARTESIAN_POINT('Ctrl Pts',(4.30000117797282,-1.36493744806469,0.652087250959406));
#13180=CARTESIAN_POINT('Ctrl Pts',(4.30000145944905,-1.36849285270534,0.645004510397983));
#13181=CARTESIAN_POINT('Ctrl Pts',(4.30000148826005,-1.36885677248754,0.644279543857467));
#13182=CARTESIAN_POINT('Ctrl Pts',(4.30000151299237,-1.36921219826683,0.643549721050429));
#13183=CARTESIAN_POINT('Ctrl Pts',(4.30000153317099,-1.36955903781249,0.642815208524159));
#13184=CARTESIAN_POINT('Ctrl Pts',(4.30000173031152,-1.37294758118467,0.635639188419686));
#13185=CARTESIAN_POINT('Ctrl Pts',(4.30000134819424,-1.37548140076902,0.628100134775109));
#13186=CARTESIAN_POINT('Ctrl Pts',(4.30000077902196,-1.37710733725971,0.620366659714886));
#13187=CARTESIAN_POINT('Ctrl Pts',(4.30000041405338,-1.37814993145247,0.615407747584041));
#13188=CARTESIAN_POINT('Ctrl Pts',(4.3,-1.37881837002099,0.610368224776708));
#13189=CARTESIAN_POINT('Ctrl Pts',(4.3,-1.37908752581626,0.605290299758539));
#13190=CARTESIAN_POINT('',(4.3,1.37908752581626,0.605290299758539));
#13191=CARTESIAN_POINT('Ctrl Pts',(4.3,1.37908752581626,0.605290299758539));
#13192=CARTESIAN_POINT('Ctrl Pts',(4.3,1.37866806817032,0.613203837240499));
#13193=CARTESIAN_POINT('Ctrl Pts',(4.30000092021544,1.37728139671899,0.621026590428679));
#13194=CARTESIAN_POINT('Ctrl Pts',(4.30000132151137,1.37501133257008,0.628597948954885));
#13195=CARTESIAN_POINT('Ctrl Pts',(4.30000154544343,1.37374458621782,0.632822935636113));
#13196=CARTESIAN_POINT('Ctrl Pts',(4.30000164013187,1.37220176226583,0.636969676056352));
#13197=CARTESIAN_POINT('Ctrl Pts',(4.30000157305315,1.37039070587839,0.641008268098125));
#13198=CARTESIAN_POINT('Ctrl Pts',(4.30000145288191,1.36714620633991,0.648243387946652));
#13199=CARTESIAN_POINT('Ctrl Pts',(4.30000073948134,1.36307905360626,0.655053358422861));
#13200=CARTESIAN_POINT('Ctrl Pts',(4.3000004635866,1.35825284513469,0.661274801567968));
#13201=CARTESIAN_POINT('Ctrl Pts',(4.30000041199046,1.35735027731582,0.662438297592388));
#13202=CARTESIAN_POINT('Ctrl Pts',(4.30000037986005,1.35642103364291,0.663581140343808));
#13203=CARTESIAN_POINT('Ctrl Pts',(4.30000037943224,1.35546536051643,0.664702144255114));
#13204=CARTESIAN_POINT('Ctrl Pts',(4.300000378582,1.3535659898678,0.666930104702213));
#13205=CARTESIAN_POINT('Ctrl Pts',(4.3000005018795,1.35156225525783,0.669071850305581));
#13206=CARTESIAN_POINT('Ctrl Pts',(4.30000067038034,1.34946148384904,0.671123623013939));
#13207=CARTESIAN_POINT('Ctrl Pts',(4.30000112630012,1.34377733881547,0.676675190215126));
#13208=CARTESIAN_POINT('Ctrl Pts',(4.30000183907902,1.33744971106208,0.68150833207295));
#13209=CARTESIAN_POINT('Ctrl Pts',(4.30000208123143,1.33064243458576,0.685568782013219));
#13210=CARTESIAN_POINT('Ctrl Pts',(4.30000223513396,1.3263159977886,0.688149444058562));
#13211=CARTESIAN_POINT('Ctrl Pts',(4.3000022300233,1.32179485563522,0.690417305529342));
#13212=CARTESIAN_POINT('Ctrl Pts',(4.30000206344016,1.31711540146937,0.692349146556373));
#13213=CARTESIAN_POINT('Ctrl Pts',(4.3000018029167,1.30979708846622,0.695370400063095));
#13214=CARTESIAN_POINT('Ctrl Pts',(4.30000114702936,1.30217656646843,0.69753735975804));
#13215=CARTESIAN_POINT('Ctrl Pts',(4.3000006156201,1.29440092269557,0.69878042986007));
#13216=CARTESIAN_POINT('Ctrl Pts',(4.30000027236218,1.28937833178082,0.699583377215073));
#13217=CARTESIAN_POINT('Ctrl Pts',(4.30000000033581,1.28429042584107,0.69999999992549));
#13218=CARTESIAN_POINT('Ctrl Pts',(4.30000000005992,1.27917501058303,0.7));
#13219=CARTESIAN_POINT('Ctrl Pts',(4.3,1.41116952203211,0.));
#13220=CARTESIAN_POINT('Ctrl Pts',(4.3,1.40583262613343,0.100695662891028));
#13221=CARTESIAN_POINT('Ctrl Pts',(4.3,1.40049561022223,0.201391319421434));
#13222=CARTESIAN_POINT('Ctrl Pts',(4.3,1.38980161287056,0.403154752748307));
#13223=CARTESIAN_POINT('Ctrl Pts',(4.3,1.38444463053604,0.504222529496425));
#13224=CARTESIAN_POINT('Ctrl Pts',(4.3,1.37908752581626,0.605290299758539));
#13225=CARTESIAN_POINT('Ctrl Pts',(4.3,-1.41116952203217,-1.08233907947231E-12));
#13226=CARTESIAN_POINT('Ctrl Pts',(4.30370667985561,-1.40059355144761,0.201807922462111));
#13227=CARTESIAN_POINT('Ctrl Pts',(4.30741340932898,-1.39001758331341,0.403615844144917));
#13228=CARTESIAN_POINT('Ctrl Pts',(4.31112018914117,-1.37944161767694,0.605423765036612));
#13229=CARTESIAN_POINT('Ctrl Pts',(3.22410085073145,-1.37636920007795,-3.90459529712038E-5));
#13230=CARTESIAN_POINT('Ctrl Pts',(3.2295286994181,-1.36579313421488,0.201768811380596));
#13231=CARTESIAN_POINT('Ctrl Pts',(3.23495659078338,-1.35521706809947,0.403576667516588));
#13232=CARTESIAN_POINT('Ctrl Pts',(3.24038452463065,-1.34464100578453,0.605384522622892));
#13233=CARTESIAN_POINT('Ctrl Pts',(2.14856196511704,-1.34935185539723,-5.92140864038068E-5));
#13234=CARTESIAN_POINT('Ctrl Pts',(2.15571155670467,-1.33877574824886,0.201748609775608));
#13235=CARTESIAN_POINT('Ctrl Pts',(2.16286118630165,-1.32819964054015,0.403556432267456));
#13236=CARTESIAN_POINT('Ctrl Pts',(2.17001085376486,-1.31762353633116,0.605364253566666));
#13237=CARTESIAN_POINT('Ctrl Pts',(1.073384157387,-1.32427529283232,-8.86713468529234E-5));
#13238=CARTESIAN_POINT('Ctrl Pts',(1.08225606990756,-1.31369916974321,0.201719104822629));
#13239=CARTESIAN_POINT('Ctrl Pts',(1.09112801825726,-1.30312304798914,0.403526879488275));
#13240=CARTESIAN_POINT('Ctrl Pts',(1.10000000295732,-1.29254692759565,0.605334652628532));
#13241=CARTESIAN_POINT('Ctrl Pts',(1.10000000298281,-1.29254692760111,0.605334652628557));
#13242=CARTESIAN_POINT('Ctrl Pts',(2.16694388170712,-1.31755402957363,0.605319894542965));
#13243=CARTESIAN_POINT('Ctrl Pts',(3.23367147240841,-1.34448060345116,0.605309774863278));
#13244=CARTESIAN_POINT('Ctrl Pts',(4.3,-1.37908752581626,0.605290299758539));
#13245=CARTESIAN_POINT('Ctrl Pts',(4.30323908112369,-1.2792801058419,0.7));
#13246=CARTESIAN_POINT('Ctrl Pts',(3.23565147654712,-1.24463335454069,0.7));
#13247=CARTESIAN_POINT('Ctrl Pts',(2.1678436779024,-1.21768649131741,0.7));
#13248=CARTESIAN_POINT('Ctrl Pts',(1.09999999999999,-1.19266190204553,0.7));
#13249=CARTESIAN_POINT('Ctrl Pts',(4.30230129178181,-1.30817667592415,0.7));
#13250=CARTESIAN_POINT('Ctrl Pts',(3.23485320804887,-1.27353066282864,0.699999860738333));
#13251=CARTESIAN_POINT('Ctrl Pts',(2.16713169816659,-1.24658393122273,0.700000105496227));
#13252=CARTESIAN_POINT('Ctrl Pts',(1.0993228455422,-1.22155728565617,0.7));
#13253=CARTESIAN_POINT('Ctrl Pts',(4.30067574076257,-1.35826558912881,0.676637683834297));
#13254=CARTESIAN_POINT('Ctrl Pts',(3.23346787205668,-1.32362126434549,0.676644071225102));
#13255=CARTESIAN_POINT('Ctrl Pts',(2.16589795861771,-1.29667457247055,0.676647306834711));
#13256=CARTESIAN_POINT('Ctrl Pts',(1.09814906228501,-1.27164470234869,0.676652147774997));
#13257=CARTESIAN_POINT('Ctrl Pts',(4.30003720890047,-1.37794098943329,0.626943772371838));
#13258=CARTESIAN_POINT('Ctrl Pts',(3.23292426239396,-1.34330449078822,0.626960286972675));
#13259=CARTESIAN_POINT('Ctrl Pts',(2.16541285690349,-1.31636171257899,0.6269687859393));
#13260=CARTESIAN_POINT('Ctrl Pts',(1.09768760301306,-1.29133598921902,0.626981304916489));
#13261=CARTESIAN_POINT('Ctrl Pts',(4.3,-1.37908752581626,0.605290299758539));
#13262=CARTESIAN_POINT('Ctrl Pts',(3.23289209128077,-1.34445530919946,0.605309789097661));
#13263=CARTESIAN_POINT('Ctrl Pts',(2.16538453588699,-1.31751467232976,0.605319909330946));
#13264=CARTESIAN_POINT('Ctrl Pts',(1.09766050997011,-1.29249209748956,0.605334684996117));
#13265=CARTESIAN_POINT('Ctrl Pts',(1.09999999999999,1.19266190204553,0.7));
#13266=CARTESIAN_POINT('Ctrl Pts',(2.1678436779024,1.21768649131741,0.7));
#13267=CARTESIAN_POINT('Ctrl Pts',(3.23565147654712,1.24463335454069,0.7));
#13268=CARTESIAN_POINT('Ctrl Pts',(4.30323908112369,1.2792801058419,0.7));
#13269=CARTESIAN_POINT('Ctrl Pts',(1.0993228455422,1.22155728565617,0.7));
#13270=CARTESIAN_POINT('Ctrl Pts',(2.16713169816659,1.24658393122273,0.700000105496227));
#13271=CARTESIAN_POINT('Ctrl Pts',(3.23485320804887,1.27353066282864,0.699999860738333));
#13272=CARTESIAN_POINT('Ctrl Pts',(4.30230129178181,1.30817667592415,0.7));
#13273=CARTESIAN_POINT('Ctrl Pts',(1.09814906228501,1.27164470234869,0.676652147774997));
#13274=CARTESIAN_POINT('Ctrl Pts',(2.16589795861771,1.29667457247055,0.676647306834711));
#13275=CARTESIAN_POINT('Ctrl Pts',(3.23346787205668,1.32362126434549,0.676644071225102));
#13276=CARTESIAN_POINT('Ctrl Pts',(4.30067574076257,1.35826558912881,0.676637683834297));
#13277=CARTESIAN_POINT('Ctrl Pts',(1.09768760301306,1.29133598921902,0.626981304916489));
#13278=CARTESIAN_POINT('Ctrl Pts',(2.16541285690349,1.31636171257899,0.6269687859393));
#13279=CARTESIAN_POINT('Ctrl Pts',(3.23292426239396,1.34330449078822,0.626960286972675));
#13280=CARTESIAN_POINT('Ctrl Pts',(4.30003720890047,1.37794098943329,0.626943772371838));
#13281=CARTESIAN_POINT('Ctrl Pts',(1.09766050997011,1.29249209748956,0.605334684996117));
#13282=CARTESIAN_POINT('Ctrl Pts',(2.16538453588699,1.31751467232976,0.605319909330946));
#13283=CARTESIAN_POINT('Ctrl Pts',(3.23289209128077,1.34445530919946,0.605309789097661));
#13284=CARTESIAN_POINT('Ctrl Pts',(4.3,1.37908752581626,0.605290299758539));
#13285=CARTESIAN_POINT('Ctrl Pts',(4.3,1.37908752581626,0.605290299758539));
#13286=CARTESIAN_POINT('Ctrl Pts',(3.23367147240841,1.34448060345116,0.605309774863278));
#13287=CARTESIAN_POINT('Ctrl Pts',(2.16694388170711,1.31755402957363,0.605319894542965));
#13288=CARTESIAN_POINT('Ctrl Pts',(1.10000000298281,1.29254692760111,0.605334652628557));
#13289=CARTESIAN_POINT('Ctrl Pts',(1.07338415738705,1.32427529283227,-8.86713457716078E-5));
#13290=CARTESIAN_POINT('Ctrl Pts',(1.08225606990759,1.31369916974318,0.201719104823349));
#13291=CARTESIAN_POINT('Ctrl Pts',(1.09112801825728,1.30312304798912,0.403526879488635));
#13292=CARTESIAN_POINT('Ctrl Pts',(1.10000000295732,1.29254692759565,0.605334652628532));
#13293=CARTESIAN_POINT('Ctrl Pts',(2.14856196511707,1.34935185539717,-5.92140853224782E-5));
#13294=CARTESIAN_POINT('Ctrl Pts',(2.15571155670469,1.33877574824882,0.201748609776328));
#13295=CARTESIAN_POINT('Ctrl Pts',(2.16286118630166,1.32819964054013,0.403556432267816));
#13296=CARTESIAN_POINT('Ctrl Pts',(2.17001085376486,1.31762353633116,0.605364253566666));
#13297=CARTESIAN_POINT('Ctrl Pts',(3.22410085073147,1.37636920007789,-3.90459518899617E-5));
#13298=CARTESIAN_POINT('Ctrl Pts',(3.22952869941811,1.36579313421484,0.201768811381317));
#13299=CARTESIAN_POINT('Ctrl Pts',(3.23495659078338,1.35521706809945,0.403576667516948));
#13300=CARTESIAN_POINT('Ctrl Pts',(3.24038452463064,1.34464100578453,0.605384522622892));
#13301=CARTESIAN_POINT('Ctrl Pts',(4.3,1.41116952203211,-1.07899800205757E-15));
#13302=CARTESIAN_POINT('Ctrl Pts',(4.3037066798556,1.40059355144758,0.201807922462832));
#13303=CARTESIAN_POINT('Ctrl Pts',(4.30741340932897,1.39001758331339,0.403615844145277));
#13304=CARTESIAN_POINT('Ctrl Pts',(4.31112018914115,1.37944161767694,0.605423765036611));
#13305=CARTESIAN_POINT('Origin',(0.9,1.39290118819044,0.));
#13306=CARTESIAN_POINT('',(0.900000001878204,-1.28788040994396,0.605337476551879));
#13307=CARTESIAN_POINT('Ctrl Pts',(0.900000001878204,-1.28788040994396,
0.605337476551879));
#13308=CARTESIAN_POINT('Ctrl Pts',(0.900000001878204,-1.29328625806092,
0.504228160928694));
#13309=CARTESIAN_POINT('Ctrl Pts',(0.899999999999999,-1.29869191435855,
0.403118132397745));
#13310=CARTESIAN_POINT('Ctrl Pts',(0.899999999999999,-1.30947917558554,
0.201339438823693));
#13311=CARTESIAN_POINT('Ctrl Pts',(0.9,-1.31486085669789,0.100669384150719));
#13312=CARTESIAN_POINT('Ctrl Pts',(0.9,-1.32024227787037,0.));
#13313=CARTESIAN_POINT('',(0.9,-1.18799600975353,0.7));
#13314=CARTESIAN_POINT('Ctrl Pts',(0.900000000000324,-1.18799600975363,
0.7));
#13315=CARTESIAN_POINT('Ctrl Pts',(0.900000000063601,-1.19590581948314,
0.699999999935493));
#13316=CARTESIAN_POINT('Ctrl Pts',(0.900000451671414,-1.20375274583281,
0.699006541951706));
#13317=CARTESIAN_POINT('Ctrl Pts',(0.900000834722547,-1.21139610511184,
0.697120084132161));
#13318=CARTESIAN_POINT('Ctrl Pts',(0.900001049758257,-1.21568690349652,
0.696061072005504));
#13319=CARTESIAN_POINT('Ctrl Pts',(0.900001241882928,-1.21991360580594,
0.694719604949841));
#13320=CARTESIAN_POINT('Ctrl Pts',(0.900001357948449,-1.22404965357203,
0.693106547509926));
#13321=CARTESIAN_POINT('Ctrl Pts',(0.900001566283472,-1.23147376710855,
0.690211145364658));
#13322=CARTESIAN_POINT('Ctrl Pts',(0.900001483882417,-1.23852542365708,
0.686475281350474));
#13323=CARTESIAN_POINT('Ctrl Pts',(0.90000115772027,-1.24505817055452,0.681980323292531));
#13324=CARTESIAN_POINT('Ctrl Pts',(0.90000097852015,-1.2486473946309,0.67951070187031));
#13325=CARTESIAN_POINT('Ctrl Pts',(0.900000731874511,-1.25207971535834,
0.676811055842604));
#13326=CARTESIAN_POINT('Ctrl Pts',(0.90000051586667,-1.25532695882913,0.673889369778116));
#13327=CARTESIAN_POINT('Ctrl Pts',(0.900000304282776,-1.25850769714062,
0.671027521295527));
#13328=CARTESIAN_POINT('Ctrl Pts',(0.900000119565725,-1.26149151526032,
0.667969976014938));
#13329=CARTESIAN_POINT('Ctrl Pts',(0.900000124706954,-1.26425564062679,
0.664728268702146));
#13330=CARTESIAN_POINT('Ctrl Pts',(0.900000134210909,-1.26936533657602,
0.658735726205464));
#13331=CARTESIAN_POINT('Ctrl Pts',(0.900000724431276,-1.2737272220214,0.652115259198653));
#13332=CARTESIAN_POINT('Ctrl Pts',(0.900000949945503,-1.27728244659665,
0.645033014705304));
#13333=CARTESIAN_POINT('Ctrl Pts',(0.900000972753073,-1.27764200720725,
0.644316745985709));
#13334=CARTESIAN_POINT('Ctrl Pts',(0.900000992743332,-1.27799327761064,
0.64359573459864));
#13335=CARTESIAN_POINT('Ctrl Pts',(0.900001009576454,-1.27833616945273,
0.642870141642621));
#13336=CARTESIAN_POINT('Ctrl Pts',(0.900001176059944,-1.28172744954266,
0.635693858502874));
#13337=CARTESIAN_POINT('Ctrl Pts',(0.900000930108723,-1.28426399347052,
0.628153947608977));
#13338=CARTESIAN_POINT('Ctrl Pts',(0.900000539908504,-1.2858931319598,0.620419547606466));
#13339=CARTESIAN_POINT('Ctrl Pts',(0.900000289636433,-1.28693805157347,
0.615458750034127));
#13340=CARTESIAN_POINT('Ctrl Pts',(0.900000000000001,-1.28760881677759,
0.610417269724172));
#13341=CARTESIAN_POINT('Ctrl Pts',(0.900000000000001,-1.28788040985668,
0.605337476551933));
#13342=CARTESIAN_POINT('',(0.9,1.18799600975353,0.7));
#13343=CARTESIAN_POINT('',(0.9,0.696450594095222,0.7));
#13344=CARTESIAN_POINT('',(0.900000001878204,1.28788040994396,0.605337476551879));
#13345=CARTESIAN_POINT('Ctrl Pts',(0.900000000000001,1.28788040985668,0.605337476551933));
#13346=CARTESIAN_POINT('Ctrl Pts',(0.900000000000001,1.28745726486871,0.613251849878237));
#13347=CARTESIAN_POINT('Ctrl Pts',(0.900000641820462,1.28606767879774,0.621075732439556));
#13348=CARTESIAN_POINT('Ctrl Pts',(0.900000906166769,1.28379497466322,0.628648019961568));
#13349=CARTESIAN_POINT('Ctrl Pts',(0.900001053446495,1.2825287445946,0.632866896498568));
#13350=CARTESIAN_POINT('Ctrl Pts',(0.900001106693909,1.28098738700664,0.637007708770872));
#13351=CARTESIAN_POINT('Ctrl Pts',(0.900001044867119,1.27917862712792,0.641040603354488));
#13352=CARTESIAN_POINT('Ctrl Pts',(0.900000933962191,1.27593407274945,0.64827481168313));
#13353=CARTESIAN_POINT('Ctrl Pts',(0.900000399592996,1.27186725264719,0.655083885116145));
#13354=CARTESIAN_POINT('Ctrl Pts',(0.900000190596867,1.2670411556595,0.661303993035384));
#13355=CARTESIAN_POINT('Ctrl Pts',(0.900000151538061,1.26613921747962,0.662466454716044));
#13356=CARTESIAN_POINT('Ctrl Pts',(0.900000126821978,1.26521063179286,0.663608275427336));
#13357=CARTESIAN_POINT('Ctrl Pts',(0.900000125264574,1.26425564063975,0.664728268702142));
#13358=CARTESIAN_POINT('Ctrl Pts',(0.90000012217056,1.26235840892454,0.66695330163032));
#13359=CARTESIAN_POINT('Ctrl Pts',(0.900000209712012,1.26035699384613,0.66909223571964));
#13360=CARTESIAN_POINT('Ctrl Pts',(0.900000331194293,1.2582587086698,0.671141334714948));
#13361=CARTESIAN_POINT('Ctrl Pts',(0.900000660246931,1.25257519443757,0.676691620936499));
#13362=CARTESIAN_POINT('Ctrl Pts',(0.900001184896248,1.24624785575673,0.681523125886843));
#13363=CARTESIAN_POINT('Ctrl Pts',(0.900001377531805,1.23944073409582,0.685581770965975));
#13364=CARTESIAN_POINT('Ctrl Pts',(0.900001499905572,1.2351164383281,0.68816006802201));
#13365=CARTESIAN_POINT('Ctrl Pts',(0.900001510509735,1.23059756718463,0.690425789971136));
#13366=CARTESIAN_POINT('Ctrl Pts',(0.900001405318139,1.22592052877826,0.692355791713551));
#13367=CARTESIAN_POINT('Ctrl Pts',(0.900001240727996,1.21860250674997,0.695375607682216));
#13368=CARTESIAN_POINT('Ctrl Pts',(0.900000792095824,1.21098234272326,0.697541065921879));
#13369=CARTESIAN_POINT('Ctrl Pts',(0.900000425437202,1.20320741268883,0.698782789564668));
#13370=CARTESIAN_POINT('Ctrl Pts',(0.900000188792485,1.19818940410026,0.699584208982791));
#13371=CARTESIAN_POINT('Ctrl Pts',(0.900000000041206,1.19310633605572,0.699999999958324));
#13372=CARTESIAN_POINT('Ctrl Pts',(0.900000000000325,1.18799600975363,0.7));
#13373=CARTESIAN_POINT('Ctrl Pts',(0.9,1.32024227787037,0.));
#13374=CARTESIAN_POINT('Ctrl Pts',(0.9,1.31486080448354,0.100670360916234));
#13375=CARTESIAN_POINT('Ctrl Pts',(0.9,1.30947907114291,0.201341392534));
#13376=CARTESIAN_POINT('Ctrl Pts',(0.9,1.2986918099064,0.403120086121531));
#13377=CARTESIAN_POINT('Ctrl Pts',(0.900000001878204,1.29328620583358,0.504229137772713));
#13378=CARTESIAN_POINT('Ctrl Pts',(0.900000001878204,1.28788040994396,0.605337476551879));
#13379=CARTESIAN_POINT('Ctrl Pts',(0.899999999999997,-1.32024227787137,
-1.86669707469278E-11));
#13380=CARTESIAN_POINT('Ctrl Pts',(0.909148787559422,-1.30966717532842,
0.201788252636133));
#13381=CARTESIAN_POINT('Ctrl Pts',(0.91829761066914,-1.29909207410335,0.403576503749508));
#13382=CARTESIAN_POINT('Ctrl Pts',(0.92744646984625,-1.28851697422138,0.605364753299354));
#13383=CARTESIAN_POINT('Ctrl Pts',(0.699273108318574,-1.31559634352334,
-5.7001548815619E-6));
#13384=CARTESIAN_POINT('Ctrl Pts',(0.708743431409066,-1.30502123870946,
0.20178254329682));
#13385=CARTESIAN_POINT('Ctrl Pts',(0.718213789763005,-1.2944461351935,0.403570785162392));
#13386=CARTESIAN_POINT('Ctrl Pts',(0.727684183892774,-1.28387103300525,
0.605359025419352));
#13387=CARTESIAN_POINT('Ctrl Pts',(0.498558799217305,-1.31100715552056,
-1.1774619888836E-5));
#13388=CARTESIAN_POINT('Ctrl Pts',(0.508350677965937,-1.30043204942944,
0.201776459055217));
#13389=CARTESIAN_POINT('Ctrl Pts',(0.518142591787393,-1.28985694462582,
0.403564691096996));
#13390=CARTESIAN_POINT('Ctrl Pts',(0.527934541191295,-1.27928184113929,
0.60535292148228));
#13391=CARTESIAN_POINT('Ctrl Pts',(0.29785707328833,-1.3064367443434,-1.84041486642056E-5));
#13392=CARTESIAN_POINT('Ctrl Pts',(0.307970527825607,-1.29586163794,0.20176981888596));
#13393=CARTESIAN_POINT('Ctrl Pts',(0.318084017341356,-1.28528653282298,
0.403558040236175));
#13394=CARTESIAN_POINT('Ctrl Pts',(0.328197542344371,-1.27471142901691,
0.605346259877786));
#13395=CARTESIAN_POINT('',(0.32957180616905,-1.2747428754212,0.605346305703265));
#13396=CARTESIAN_POINT('Ctrl Pts',(0.297857995688647,-1.306435779838,1.57426155444895E-16));
#13397=CARTESIAN_POINT('Ctrl Pts',(0.308429283449307,-1.29587142805659,
0.201782098465301));
#13398=CARTESIAN_POINT('Ctrl Pts',(0.319000553694994,-1.28530712634462,
0.403564200350135));
#13399=CARTESIAN_POINT('Ctrl Pts',(0.329571806169048,-1.2747428754212,0.605346305703266));
#13400=CARTESIAN_POINT('Ctrl Pts',(0.32957180616905,-1.2747428754212,0.605346305703265));
#13401=CARTESIAN_POINT('Ctrl Pts',(0.519721397561595,-1.27909449722757,
0.60534313598158));
#13402=CARTESIAN_POINT('Ctrl Pts',(0.709864288600121,-1.28346276435313,
0.605340219076093));
#13403=CARTESIAN_POINT('Ctrl Pts',(0.900000001879218,-1.28788040990034,
0.605337476551906));
#13404=CARTESIAN_POINT('Ctrl Pts',(0.90231940407953,-1.18804989493878,0.7));
#13405=CARTESIAN_POINT('Ctrl Pts',(0.712166351817731,-1.18363199317816,
0.7));
#13406=CARTESIAN_POINT('Ctrl Pts',(0.522011847238247,-1.17926361631973,
0.7));
#13407=CARTESIAN_POINT('Ctrl Pts',(0.331856371369203,-1.17491202960101,
0.7));
#13408=CARTESIAN_POINT('Ctrl Pts',(0.901648075315333,-1.21694488185794,
0.7));
#13409=CARTESIAN_POINT('Ctrl Pts',(0.711500071980331,-1.21252656425213,
0.69999998041973));
#13410=CARTESIAN_POINT('Ctrl Pts',(0.521348914609444,-1.20815772874132,
0.700000022626678));
#13411=CARTESIAN_POINT('Ctrl Pts',(0.331195161244126,-1.20380556524924,
0.7));
#13412=CARTESIAN_POINT('Ctrl Pts',(0.900484091294294,-1.26704448261357,
0.676664431332699));
#13413=CARTESIAN_POINT('Ctrl Pts',(0.710344780071471,-1.26262550764723,
0.676665329845182));
#13414=CARTESIAN_POINT('Ctrl Pts',(0.520199507967113,-1.25825584722226,
0.676666267597974));
#13415=CARTESIAN_POINT('Ctrl Pts',(0.3300487189482,-1.25390275839508,0.676667306001616));
#13416=CARTESIAN_POINT('Ctrl Pts',(0.90002687589075,-1.28672371253673,0.626983665342106));
#13417=CARTESIAN_POINT('Ctrl Pts',(0.709890987426059,-1.28230548388611,
0.626985988983916));
#13418=CARTESIAN_POINT('Ctrl Pts',(0.519747959090447,-1.27793661492756,
0.626988445273931));
#13419=CARTESIAN_POINT('Ctrl Pts',(0.329598318905021,-1.27358432286302,
0.626991130804315));
#13420=CARTESIAN_POINT('Ctrl Pts',(0.900000001879218,-1.28788040990034,
0.605337476551906));
#13421=CARTESIAN_POINT('Ctrl Pts',(0.709864288600121,-1.28346276435313,
0.605340219076093));
#13422=CARTESIAN_POINT('Ctrl Pts',(0.519721397561595,-1.27909449722757,
0.60534313598158));
#13423=CARTESIAN_POINT('Ctrl Pts',(0.32957180616905,-1.2747428754212,0.605346305703265));
#13424=CARTESIAN_POINT('',(0.331856371369201,-1.17491202962433,0.7));
#13425=CARTESIAN_POINT('Origin',(0.331856371539144,-1.1749120296049,0.6));
#13426=CARTESIAN_POINT('Ctrl Pts',(0.900000000000328,-1.18799600975363,
0.7));
#13427=CARTESIAN_POINT('Ctrl Pts',(0.71062007065371,-1.18359647108512,0.7));
#13428=CARTESIAN_POINT('Ctrl Pts',(0.521238702715143,-1.17924592340069,
0.7));
#13429=CARTESIAN_POINT('Ctrl Pts',(0.331856371369203,-1.17491202960101,
0.7));
#13430=CARTESIAN_POINT('Origin',(6.87409734069396,-2.22251806091942E-16,
0.7));
#13431=CARTESIAN_POINT('',(0.331856371879032,1.17491202961268,0.7));
#13432=CARTESIAN_POINT('',(0.331856371369201,-0.75,0.7));
#13433=CARTESIAN_POINT('Ctrl Pts',(0.331856371879031,1.17491202961268,0.7));
#13434=CARTESIAN_POINT('Ctrl Pts',(0.521238703055026,1.1792459234085,0.7));
#13435=CARTESIAN_POINT('Ctrl Pts',(0.710620070823648,1.18359647108907,0.7));
#13436=CARTESIAN_POINT('Ctrl Pts',(0.900000000000325,1.18799600975363,0.7));
#13437=CARTESIAN_POINT('Ctrl Pts',(0.297857073289265,1.30643674434242,-1.84041299971672E-5));
#13438=CARTESIAN_POINT('Ctrl Pts',(0.30797052782623,1.29586163793935,0.201769818898405));
#13439=CARTESIAN_POINT('Ctrl Pts',(0.318084017341667,1.28528653282265,0.403558040242397));
#13440=CARTESIAN_POINT('Ctrl Pts',(0.328197542344371,1.27471142901691,0.605346259877786));
#13441=CARTESIAN_POINT('Ctrl Pts',(0.49855879921793,1.31100715551957,-1.17746012218085E-5));
#13442=CARTESIAN_POINT('Ctrl Pts',(0.50835067796626,1.30043204942878,0.201776459067662));
#13443=CARTESIAN_POINT('Ctrl Pts',(0.518142591787414,1.28985694462549,0.403564691103219));
#13444=CARTESIAN_POINT('Ctrl Pts',(0.527934541191015,1.27928184113928,0.60535292148228));
#13445=CARTESIAN_POINT('Ctrl Pts',(0.699273108318888,1.31559634352235,-5.70013621459206E-6));
#13446=CARTESIAN_POINT('Ctrl Pts',(0.708743431409089,1.3050212387088,0.201782543309265));
#13447=CARTESIAN_POINT('Ctrl Pts',(0.718213789762737,1.29444613519316,0.403570785168614));
#13448=CARTESIAN_POINT('Ctrl Pts',(0.727684183892215,1.28387103300524,0.605359025419352));
#13449=CARTESIAN_POINT('Ctrl Pts',(0.9,1.32024227787037,-6.93889390390723E-18));
#13450=CARTESIAN_POINT('Ctrl Pts',(0.909148787559144,1.30966717532775,0.201788252648578));
#13451=CARTESIAN_POINT('Ctrl Pts',(0.918297610668582,1.29909207410301,0.403576503755731));
#13452=CARTESIAN_POINT('Ctrl Pts',(0.927446469845411,1.28851697422136,0.605364753299355));
#13453=CARTESIAN_POINT('',(0.329571806169048,1.2747428754212,0.605346305703265));
#13454=CARTESIAN_POINT('Ctrl Pts',(0.900000001879216,1.28788040990034,0.605337476551906));
#13455=CARTESIAN_POINT('Ctrl Pts',(0.709864288600119,1.28346276435313,0.605340219076093));
#13456=CARTESIAN_POINT('Ctrl Pts',(0.519721397561593,1.27909449722757,0.60534313598158));
#13457=CARTESIAN_POINT('Ctrl Pts',(0.329571806169048,1.2747428754212,0.605346305703265));
#13458=CARTESIAN_POINT('Ctrl Pts',(0.329571806169048,1.2747428754212,0.605346305703265));
#13459=CARTESIAN_POINT('Ctrl Pts',(0.319000553694994,1.28530712634462,0.403564200350134));
#13460=CARTESIAN_POINT('Ctrl Pts',(0.308429283449307,1.29587142805659,0.201782098465301));
#13461=CARTESIAN_POINT('Ctrl Pts',(0.297857995688647,1.306435779838,6.03900610074426E-17));
#13462=CARTESIAN_POINT('Ctrl Pts',(0.331856371369201,1.17491202960101,0.7));
#13463=CARTESIAN_POINT('Ctrl Pts',(0.522011847238246,1.17926361631973,0.7));
#13464=CARTESIAN_POINT('Ctrl Pts',(0.712166351817729,1.18363199317816,0.7));
#13465=CARTESIAN_POINT('Ctrl Pts',(0.902319404079528,1.18804989493878,0.7));
#13466=CARTESIAN_POINT('Ctrl Pts',(0.331195161244124,1.20380556524924,0.7));
#13467=CARTESIAN_POINT('Ctrl Pts',(0.521348914609443,1.20815772874132,0.700000022626678));
#13468=CARTESIAN_POINT('Ctrl Pts',(0.711500071980329,1.21252656425213,0.69999998041973));
#13469=CARTESIAN_POINT('Ctrl Pts',(0.901648075315331,1.21694488185794,0.7));
#13470=CARTESIAN_POINT('Ctrl Pts',(0.330048718948197,1.25390275839508,0.676667306001616));
#13471=CARTESIAN_POINT('Ctrl Pts',(0.52019950796711,1.25825584722226,0.676666267597973));
#13472=CARTESIAN_POINT('Ctrl Pts',(0.710344780071469,1.26262550764723,0.676665329845182));
#13473=CARTESIAN_POINT('Ctrl Pts',(0.900484091294292,1.26704448261357,0.676664431332698));
#13474=CARTESIAN_POINT('Ctrl Pts',(0.329598318905018,1.27358432286302,0.626991130804315));
#13475=CARTESIAN_POINT('Ctrl Pts',(0.519747959090446,1.27793661492756,0.62698844527393));
#13476=CARTESIAN_POINT('Ctrl Pts',(0.709890987426057,1.28230548388611,0.626985988983916));
#13477=CARTESIAN_POINT('Ctrl Pts',(0.900026875890748,1.28672371253673,0.626983665342106));
#13478=CARTESIAN_POINT('Ctrl Pts',(0.329571806169048,1.2747428754212,0.605346305703265));
#13479=CARTESIAN_POINT('Ctrl Pts',(0.519721397561593,1.27909449722757,0.60534313598158));
#13480=CARTESIAN_POINT('Ctrl Pts',(0.709864288600119,1.28346276435313,0.605340219076093));
#13481=CARTESIAN_POINT('Ctrl Pts',(0.900000001879216,1.28788040990034,0.605337476551906));
#13482=CARTESIAN_POINT('Origin',(0.331856371369202,1.17491202960101,0.6));
#13483=CARTESIAN_POINT('Origin',(0.331856371369202,1.17491202960101,0.6));
#13484=CARTESIAN_POINT('Origin',(0.331856371369201,1.17491202960879,0.6));
#13485=CARTESIAN_POINT('Origin',(0.331856371369202,1.17491202960101,0.6));
#13486=CARTESIAN_POINT('Origin',(12.8681436286308,1.83274446434879,0.6));
#13487=CARTESIAN_POINT('Origin',(12.8681436286308,1.83274446434879,0.6));
#13488=CARTESIAN_POINT('',(12.9680065821063,1.83274446434879,0.605233595624294));
#13489=CARTESIAN_POINT('Origin',(12.8681436286308,1.83274446434879,0.6));
#13490=CARTESIAN_POINT('Origin',(12.8681436286308,1.83274446434879,0.6));
#13491=CARTESIAN_POINT('Origin',(0.331856371369201,-1.17491202960101,0.6));
#13492=CARTESIAN_POINT('Origin',(0.331856371369201,-1.17491202960101,0.6));
#13493=CARTESIAN_POINT('Origin',(0.331856371369201,-1.17491202960101,0.6));
#13494=CARTESIAN_POINT('Origin',(0.331856371369201,-0.75,0.6));
#13495=CARTESIAN_POINT('Ctrl Pts',(0.297750759617602,-1.30654294555098,
-0.00204689530870639));
#13496=CARTESIAN_POINT('Ctrl Pts',(0.308357792853923,-1.29594287152607,
0.200417501569666));
#13497=CARTESIAN_POINT('Ctrl Pts',(0.318964808457496,-1.28534284790734,
0.40288190189057));
#13498=CARTESIAN_POINT('Ctrl Pts',(0.329571806169048,-1.2747428754212,0.605346305703266));
#13499=CARTESIAN_POINT('Ctrl Pts',(0.268364475985512,-1.30579334864515,
-0.000546070465277405));
#13500=CARTESIAN_POINT('Ctrl Pts',(0.278972236061358,-1.29519218153762,
0.201918231169276));
#13501=CARTESIAN_POINT('Ctrl Pts',(0.289579970322816,-1.28459115545203,
0.404382541571378));
#13502=CARTESIAN_POINT('Ctrl Pts',(0.300187702091134,-1.27399007937578,
0.606846849214128));
#13503=CARTESIAN_POINT('Ctrl Pts',(0.217994620733579,-1.28028753054242,
0.000758348866131992));
#13504=CARTESIAN_POINT('Ctrl Pts',(0.228604439653725,-1.26968580576698,
0.203222517770204));
#13505=CARTESIAN_POINT('Ctrl Pts',(0.239214264875756,-1.259084092946,0.405686686833815));
#13506=CARTESIAN_POINT('Ctrl Pts',(0.24982407554016,-1.24848245399652,0.608150860486448));
#13507=CARTESIAN_POINT('Ctrl Pts',(0.200221638751335,-1.22875730734246,
-0.00100806500432267));
#13508=CARTESIAN_POINT('Ctrl Pts',(0.210832346469089,-1.21815680658782,
0.201456130081263));
#13509=CARTESIAN_POINT('Ctrl Pts',(0.221443027663539,-1.20755634130466,
0.403920328365886));
#13510=CARTESIAN_POINT('Ctrl Pts',(0.232053735729819,-1.1969559383274,0.606384528499152));
#13511=CARTESIAN_POINT('Ctrl Pts',(0.200161316008396,-1.20671181983024,
-0.00215909150772397));
#13512=CARTESIAN_POINT('Ctrl Pts',(0.21077201649647,-1.19611183845239,0.200305134857769));
#13513=CARTESIAN_POINT('Ctrl Pts',(0.221382717124246,-1.18551190812967,
0.402769363888924));
#13514=CARTESIAN_POINT('Ctrl Pts',(0.231993417893744,-1.17491202960101,
0.605233595624295));
#13515=CARTESIAN_POINT('Origin',(12.8681436286308,-1.83274446434879,0.6));
#13516=CARTESIAN_POINT('',(12.9680065821063,-1.83274446434879,0.605233595624295));
#13517=CARTESIAN_POINT('Origin',(12.8681436286308,-1.83274446434879,0.6));
#13518=CARTESIAN_POINT('Origin',(12.8681436286308,-1.83274446434879,0.6));
#13519=CARTESIAN_POINT('Origin',(12.8681436286308,1.1,0.6));
#13520=CARTESIAN_POINT('',(12.9680065821063,1.1,0.605233595624295));
#13521=CARTESIAN_POINT('Ctrl Pts',(12.9998428721614,-1.86475648739599,-0.00223900654757928));
#13522=CARTESIAN_POINT('Ctrl Pts',(12.9892307746816,-1.85408610159386,0.200251876006837));
#13523=CARTESIAN_POINT('Ctrl Pts',(12.9786186779927,-1.84341542867022,0.402742743472647));
#13524=CARTESIAN_POINT('Ctrl Pts',(12.9680065821063,-1.83274446434879,0.605233595624296));
#13525=CARTESIAN_POINT('Ctrl Pts',(12.9997989521977,-1.88070362541494,-0.00140096371806573));
#13526=CARTESIAN_POINT('Ctrl Pts',(12.9891868560404,-1.87003481788623,0.2010900171988));
#13527=CARTESIAN_POINT('Ctrl Pts',(12.9785747412344,-1.85936572080465,0.403580981971657));
#13528=CARTESIAN_POINT('Ctrl Pts',(12.967962646681,-1.84869634914788,0.606071933479074));
#13529=CARTESIAN_POINT('Ctrl Pts',(12.9919061104719,-1.91252097257855,-0.00013797468654593));
#13530=CARTESIAN_POINT('Ctrl Pts',(12.9812924311808,-1.9018552985481,0.202353118580234));
#13531=CARTESIAN_POINT('Ctrl Pts',(12.970678744243,-1.89118929884075,0.404844194499128));
#13532=CARTESIAN_POINT('Ctrl Pts',(12.9600650516023,-1.88052308923615,0.607335259545336));
#13533=CARTESIAN_POINT('Ctrl Pts',(12.9539932318948,-1.95585643963679,0.000158685530800887));
#13534=CARTESIAN_POINT('Ctrl Pts',(12.9433725220626,-1.94519261899951,0.202649549046396));
#13535=CARTESIAN_POINT('Ctrl Pts',(12.9327517623504,-1.93452853669393,0.40514039680648));
#13536=CARTESIAN_POINT('Ctrl Pts',(12.9221309734579,-1.92386419524738,0.607631230057729));
#13537=CARTESIAN_POINT('Ctrl Pts',(12.9129235702791,-1.96658826742031,-0.00142816374191492));
#13538=CARTESIAN_POINT('Ctrl Pts',(12.9022969271978,-1.95592037993921,0.201062184830579));
#13539=CARTESIAN_POINT('Ctrl Pts',(12.891670251582,-1.94525202616943,0.403552507423554));
#13540=CARTESIAN_POINT('Ctrl Pts',(12.8810434760214,-1.93458357684419,0.60604282089977));
#13541=CARTESIAN_POINT('Ctrl Pts',(12.8891437477602,-1.96405813112492,-0.00280773857265357));
#13542=CARTESIAN_POINT('Ctrl Pts',(12.8785151960038,-1.95338599020215,0.199682283294402));
#13543=CARTESIAN_POINT('Ctrl Pts',(12.8678865709412,-1.94271355010484,0.402172286243574));
#13544=CARTESIAN_POINT('Ctrl Pts',(12.8572578715866,-1.93204080633595,0.604662269998931));
#13545=CARTESIAN_POINT('Ctrl Pts',(12.9997255308004,-1.86463850151065,-4.9439619065339E-17));
#13546=CARTESIAN_POINT('Ctrl Pts',(12.9891525471135,-1.85400744222428,0.201744546927532));
#13547=CARTESIAN_POINT('Ctrl Pts',(12.9785795642115,-1.84337609791338,0.403489078876654));
#13548=CARTESIAN_POINT('Ctrl Pts',(12.9680065821063,-1.83274446434879,0.605233595624296));
#13549=CARTESIAN_POINT('Ctrl Pts',(12.8891409639924,1.96405533594058,-0.00275470357795049));
#13550=CARTESIAN_POINT('Ctrl Pts',(12.8785133401458,1.95338412669368,0.199717639954231));
#13551=CARTESIAN_POINT('Ctrl Pts',(12.8678856430057,1.9427126183241,0.402189964571813));
#13552=CARTESIAN_POINT('Ctrl Pts',(12.8572578715866,1.93204080633595,0.604662269998929));
#13553=CARTESIAN_POINT('Ctrl Pts',(12.9049941793403,1.96574209420267,-0.00183498696757459));
#13554=CARTESIAN_POINT('Ctrl Pts',(12.8943678341644,1.95507368670196,0.20063757283533));
#13555=CARTESIAN_POINT('Ctrl Pts',(12.8837414238008,1.94440496992476,0.403110113573296));
#13556=CARTESIAN_POINT('Ctrl Pts',(12.8731149412098,1.93373598667478,0.605582637266155));
#13557=CARTESIAN_POINT('Ctrl Pts',(12.9374710816243,1.9613461313261,-0.000364592700753267));
#13558=CARTESIAN_POINT('Ctrl Pts',(12.9268487371951,1.95068187676899,0.202108391447626));
#13559=CARTESIAN_POINT('Ctrl Pts',(12.9162262930262,1.94001732715406,0.404581355450702));
#13560=CARTESIAN_POINT('Ctrl Pts',(12.9056038462248,1.92935253789361,0.607054307450502));
#13561=CARTESIAN_POINT('Ctrl Pts',(12.9846523118271,1.92834870343354,0.000369250346899581));
#13562=CARTESIAN_POINT('Ctrl Pts',(12.974038022963,1.91768545846127,0.202842678583437));
#13563=CARTESIAN_POINT('Ctrl Pts',(12.9634237233674,1.90702194269714,0.405316092420461));
#13564=CARTESIAN_POINT('Ctrl Pts',(12.9528094065597,1.89635817580376,0.607789492622546));
#13565=CARTESIAN_POINT('Ctrl Pts',(12.9997742127558,1.88867440031858,-0.000928907044737527));
#13566=CARTESIAN_POINT('Ctrl Pts',(12.9891630904765,1.8780073281596,0.201544447891303));
#13567=CARTESIAN_POINT('Ctrl Pts',(12.9785517991681,1.86733992038445,0.404017776344753));
#13568=CARTESIAN_POINT('Ctrl Pts',(12.9679406789684,1.85667229154743,0.606491102406462));
#13569=CARTESIAN_POINT('Ctrl Pts',(12.9998400927033,1.86475369267134,-0.00218597132744988));
#13570=CARTESIAN_POINT('Ctrl Pts',(12.9892289217097,1.85408423839396,0.200287232817622));
#13571=CARTESIAN_POINT('Ctrl Pts',(12.9786177515068,1.84341449704483,0.402760421876702));
#13572=CARTESIAN_POINT('Ctrl Pts',(12.9680065821063,1.83274446434879,0.605233595624294));
#13573=CARTESIAN_POINT('Ctrl Pts',(12.9680065821063,1.83274446434879,0.605233595624294));
#13574=CARTESIAN_POINT('Ctrl Pts',(12.9785795642115,1.84337609791338,0.403489078876654));
#13575=CARTESIAN_POINT('Ctrl Pts',(12.9891525471135,1.85400744222428,0.201744546927532));
#13576=CARTESIAN_POINT('Ctrl Pts',(12.9997255308004,1.86463850151065,1.86916454536501E-16));
#13577=CARTESIAN_POINT('Ctrl Pts',(12.6,1.80383022254432,0.7));
#13578=CARTESIAN_POINT('Ctrl Pts',(12.6893984576578,1.8133105623702,0.7));
#13579=CARTESIAN_POINT('Ctrl Pts',(12.7787800350189,1.82294762441299,0.7));
#13580=CARTESIAN_POINT('Ctrl Pts',(12.8681436286308,1.83274446434879,0.7));
#13581=CARTESIAN_POINT('Ctrl Pts',(12.5969393303222,1.83269196733649,0.7));
#13582=CARTESIAN_POINT('Ctrl Pts',(12.686303642571,1.84217134991284,0.700000098415946));
#13583=CARTESIAN_POINT('Ctrl Pts',(12.7756511334299,1.85180730951691,0.699999896874207));
#13584=CARTESIAN_POINT('Ctrl Pts',(12.8649798835675,1.86160311979107,0.7));
#13585=CARTESIAN_POINT('Ctrl Pts',(12.5916356538948,1.88270499442536,0.67643906321291));
#13586=CARTESIAN_POINT('Ctrl Pts',(12.6809412203008,1.89218243450198,0.676434576658958));
#13587=CARTESIAN_POINT('Ctrl Pts',(12.7702288461642,1.90181652272411,0.676430055978541));
#13588=CARTESIAN_POINT('Ctrl Pts',(12.8594976525144,1.91161025179704,0.676425356750174));
#13589=CARTESIAN_POINT('Ctrl Pts',(12.58957419749,1.90214427893475,0.626447702441804));
#13590=CARTESIAN_POINT('Ctrl Pts',(12.6788572782758,1.91161594713488,0.626436135819418));
#13591=CARTESIAN_POINT('Ctrl Pts',(12.7681225846323,1.92124403769089,0.626424372515079));
#13592=CARTESIAN_POINT('Ctrl Pts',(12.8573684983393,1.93103170500986,0.626412260100396));
#13593=CARTESIAN_POINT('Ctrl Pts',(12.5894662143615,1.90316254677271,0.604704117718382));
#13594=CARTESIAN_POINT('Ctrl Pts',(12.6787484942245,1.91263121188366,0.60469048808123));
#13595=CARTESIAN_POINT('Ctrl Pts',(12.7680127446979,1.92225628370762,0.604676541242762));
#13596=CARTESIAN_POINT('Ctrl Pts',(12.8572578715866,1.93204080633595,0.60466226999893));
#13597=CARTESIAN_POINT('Ctrl Pts',(0.200160815981423,1.20671231935208,-0.00216863259073552));
#13598=CARTESIAN_POINT('Ctrl Pts',(0.21077168314515,1.19611217146534,0.200298774135678));
#13599=CARTESIAN_POINT('Ctrl Pts',(0.221382550448584,1.18551207463533,0.402766183527835));
#13600=CARTESIAN_POINT('Ctrl Pts',(0.231993417893744,1.17491202960101,0.605233595624295));
#13601=CARTESIAN_POINT('Ctrl Pts',(0.200241246305444,1.23610630273461,-0.000633930584249493));
#13602=CARTESIAN_POINT('Ctrl Pts',(0.210852138766318,1.22550544237485,0.201833432539687));
#13603=CARTESIAN_POINT('Ctrl Pts',(0.221462948692539,1.21490467236247,0.404300804744641));
#13604=CARTESIAN_POINT('Ctrl Pts',(0.232073841675177,1.20430390790287,0.60676817279077));
#13605=CARTESIAN_POINT('Ctrl Pts',(0.224595236946023,1.28704077752974,0.000756396927320467));
#13606=CARTESIAN_POINT('Ctrl Pts',(0.235204871724134,1.27643877611169,0.203223757667495));
#13607=CARTESIAN_POINT('Ctrl Pts',(0.245814524913363,1.26583679641595,0.405691118453359));
#13608=CARTESIAN_POINT('Ctrl Pts',(0.256424148042823,1.25523487973404,0.608158484046399));
#13609=CARTESIAN_POINT('Ctrl Pts',(0.275710547013829,1.30598124743532,-0.000930817763883136));
#13610=CARTESIAN_POINT('Ctrl Pts',(0.286318282165364,1.29538020346814,0.201536689442792));
#13611=CARTESIAN_POINT('Ctrl Pts',(0.296926023167072,1.2847792285374,0.404004199876323));
#13612=CARTESIAN_POINT('Ctrl Pts',(0.307533728110612,1.27417827838713,0.606471713336412));
#13613=CARTESIAN_POINT('Ctrl Pts',(0.297750259763447,1.30654344507719,-0.0020564363997533));
#13614=CARTESIAN_POINT('Ctrl Pts',(0.308357459618374,1.29594320454196,0.200411140842193));
#13615=CARTESIAN_POINT('Ctrl Pts',(0.318964641840002,1.28534301441448,0.402878721526778));
#13616=CARTESIAN_POINT('Ctrl Pts',(0.329571806169048,1.2747428754212,0.605346305703265));
#13617=CARTESIAN_POINT('Origin',(13.0002740930491,2.2,-0.0104671912485888));
#13618=CARTESIAN_POINT('Origin',(0.331856371369202,1.17491202960101,0.6));
#13619=CARTESIAN_POINT('',(0.331856371879032,1.17491202961268,0.9));
#13620=CARTESIAN_POINT('',(0.0322675109428289,1.17491202960101,0.615700786872883));
#13621=CARTESIAN_POINT('Origin',(0.331856371369201,1.17491202962433,0.6));
#13622=CARTESIAN_POINT('',(0.325002675768741,1.47440456706157,0.616038917109795));
#13623=CARTESIAN_POINT('Origin',(0.331856371369202,1.17491202960101,0.6));
#13624=CARTESIAN_POINT('Origin',(0.331856371369201,1.17491202960101,0.6));
#13625=CARTESIAN_POINT('Origin',(12.8681436286308,1.83274446434879,0.6));
#13626=CARTESIAN_POINT('',(12.8681436286308,1.83274446434879,0.9));
#13627=CARTESIAN_POINT('',(12.8354863574981,2.13063349031027,0.613986809996789));
#13628=CARTESIAN_POINT('Origin',(12.8681436286308,1.83274446434879,0.6));
#13629=CARTESIAN_POINT('',(13.1677324890572,1.83274446434879,0.615700786872883));
#13630=CARTESIAN_POINT('Origin',(12.8681436286308,1.83274446434879,0.6));
#13631=CARTESIAN_POINT('Origin',(12.8681436286308,1.83274446434879,0.6));
#13632=CARTESIAN_POINT('Origin',(0.331856371369201,-1.17491202960101,0.6));
#13633=CARTESIAN_POINT('',(0.331856371369201,-1.17491202962433,0.9));
#13634=CARTESIAN_POINT('',(0.325002675768743,-1.47440456706157,0.616038917109795));
#13635=CARTESIAN_POINT('Origin',(0.331856371879032,-1.17491202961268,0.6));
#13636=CARTESIAN_POINT('',(0.0322675109428289,-1.17491202960101,0.615700786872884));
#13637=CARTESIAN_POINT('Origin',(0.331856371369201,-1.17491202960101,0.6));
#13638=CARTESIAN_POINT('Origin',(0.331856371369201,-1.17491202960101,0.6));
#13639=CARTESIAN_POINT('Origin',(0.331856371369201,-0.75,0.6));
#13640=CARTESIAN_POINT('',(0.0322675109428289,-0.75,0.615700786872883));
#13641=CARTESIAN_POINT('',(0.331856371369201,-0.75,0.9));
#13642=CARTESIAN_POINT('Ctrl Pts',(0.292429673212981,-1.5069793045954,-0.00614074949474724));
#13643=CARTESIAN_POINT('Ctrl Pts',(0.303287396789886,-1.49612100698918,
0.201252467440773));
#13644=CARTESIAN_POINT('Ctrl Pts',(0.314145064588525,-1.48526276089333,
0.408645689616972));
#13645=CARTESIAN_POINT('Ctrl Pts',(0.325002675768741,-1.47440456706157,
0.616038917109795));
#13646=CARTESIAN_POINT('Ctrl Pts',(0.204270663953122,-1.50473074636003,
-0.00163825452108868));
#13647=CARTESIAN_POINT('Ctrl Pts',(0.215130619942527,-1.49386909866124,
0.205754670272474));
#13648=CARTESIAN_POINT('Ctrl Pts',(0.225990497234893,-1.48300775583971,
0.413147615201549));
#13649=CARTESIAN_POINT('Ctrl Pts',(0.236850363534999,-1.47214617892531,
0.620540547642382));
#13650=CARTESIAN_POINT('Ctrl Pts',(0.0531014592841718,-1.42831231122466,
0.00228331220810075));
#13651=CARTESIAN_POINT('Ctrl Pts',(0.0639677431943945,-1.41744892560022,
0.209675827753147));
#13652=CARTESIAN_POINT('Ctrl Pts',(0.0748340498672138,-1.40658548887187,
0.417068339030394));
#13653=CARTESIAN_POINT('Ctrl Pts',(0.0857003072238147,-1.3957221574093,
0.624460858243749));
#13654=CARTESIAN_POINT('Ctrl Pts',(-0.000158492362241063,-1.27362248439808,
-0.0030242144278773));
#13655=CARTESIAN_POINT('Ctrl Pts',(0.0107105192099893,-1.2627628846508,
0.204368383073371));
#13656=CARTESIAN_POINT('Ctrl Pts',(0.0215794523842628,-1.25190326350425,
0.411760983371354));
#13657=CARTESIAN_POINT('Ctrl Pts',(0.0324484644510542,-1.24104375578019,
0.619153585497454));
#13658=CARTESIAN_POINT('Ctrl Pts',(-0.000339460947516079,-1.20748590713937,
-0.00647730073969574));
#13659=CARTESIAN_POINT('Ctrl Pts',(0.0105295295353408,-1.19662789414299,
0.200915392321314));
#13660=CARTESIAN_POINT('Ctrl Pts',(0.0213985201647323,-1.18576993469886,
0.408308088178364));
#13661=CARTESIAN_POINT('Ctrl Pts',(0.032267510942829,-1.17491202960101,
0.615700786872884));
#13662=CARTESIAN_POINT('Ctrl Pts',(0.292751161823634,-1.50665779898694,
4.33680868994202E-17));
#13663=CARTESIAN_POINT('Ctrl Pts',(0.30350172143464,-1.49590667092872,0.205346300540216));
#13664=CARTESIAN_POINT('Ctrl Pts',(0.314252226354851,-1.48515559337638,
0.410692606218909));
#13665=CARTESIAN_POINT('Ctrl Pts',(0.325002675768741,-1.47440456706157,
0.616038917109795));
#13666=CARTESIAN_POINT('Ctrl Pts',(0.032267510942829,-1.17491202960101,
0.615700786872884));
#13667=CARTESIAN_POINT('Ctrl Pts',(0.021511673816962,-1.18565689645617,
0.410467188483275));
#13668=CARTESIAN_POINT('Ctrl Pts',(0.0107558368367201,-1.19640181653194,
0.205233592872363));
#13669=CARTESIAN_POINT('Ctrl Pts',(-2.19605150036939E-16,-1.20714678905882,
1.11889664200504E-16));
#13670=CARTESIAN_POINT('Origin',(12.8681436286308,-1.83274446434879,0.6));
#13671=CARTESIAN_POINT('',(13.1677324890572,-1.83274446434879,0.615700786872883));
#13672=CARTESIAN_POINT('',(12.8354863574981,-2.13063349031027,0.613986809996789));
#13673=CARTESIAN_POINT('Origin',(12.8681436286308,-1.83274446434879,0.6));
#13674=CARTESIAN_POINT('',(12.8681436286308,-1.83274446434879,0.9));
#13675=CARTESIAN_POINT('Origin',(12.8681436286308,-1.83274446434879,0.6));
#13676=CARTESIAN_POINT('Origin',(12.8681436286308,-1.83274446434879,0.6));
#13677=CARTESIAN_POINT('Origin',(12.8681436286308,1.1,0.6));
#13678=CARTESIAN_POINT('',(13.1677324890572,1.1,0.615700786872883));
#13679=CARTESIAN_POINT('',(12.8681436286308,1.1,0.9));
#13680=CARTESIAN_POINT('Ctrl Pts',(12.8681436286308,-1.83274446434879,0.9));
#13681=CARTESIAN_POINT('Ctrl Pts',(11.0848390724976,-1.63724259846481,0.9));
#13682=CARTESIAN_POINT('Ctrl Pts',(6.90843812479705,-1.33014681916253,0.9));
#13683=CARTESIAN_POINT('Ctrl Pts',(2.72316671642812,-1.22963564084767,0.9));
#13684=CARTESIAN_POINT('Ctrl Pts',(0.331856371369203,-1.17491202960101,
0.9));
#13685=CARTESIAN_POINT('Ctrl Pts',(12.8586523934408,-1.91932043067563,0.9));
#13686=CARTESIAN_POINT('Ctrl Pts',(11.0774332085042,-1.7238803779394,0.89999435405169));
#13687=CARTESIAN_POINT('Ctrl Pts',(6.90489492800773,-1.41683381760594,0.900002805573959));
#13688=CARTESIAN_POINT('Ctrl Pts',(2.72111811994416,-1.31633797570969,0.90000078069347));
#13689=CARTESIAN_POINT('Ctrl Pts',(0.329872740993971,-1.26159263654569,
0.9));
#13690=CARTESIAN_POINT('Ctrl Pts',(12.8422006781022,-2.06938763738452,0.829321796184829));
#13691=CARTESIAN_POINT('Ctrl Pts',(11.0645720435655,-1.87407163985848,0.829602081442736));
#13692=CARTESIAN_POINT('Ctrl Pts',(6.89876476423634,-1.56711486110062,0.829953500700133));
#13693=CARTESIAN_POINT('Ctrl Pts',(2.71756729604702,-1.46664725828863,0.829952661937692));
#13694=CARTESIAN_POINT('Ctrl Pts',(0.326433810179884,-1.41186690836963,
0.829991693349937));
#13695=CARTESIAN_POINT('Ctrl Pts',(12.8358182377562,-2.12760618633201,0.679236780301187));
#13696=CARTESIAN_POINT('Ctrl Pts',(11.0595580661442,-1.93265366192027,0.679962478070753));
#13697=CARTESIAN_POINT('Ctrl Pts',(6.89634818471837,-1.62613750062048,0.680874066334139));
#13698=CARTESIAN_POINT('Ctrl Pts',(2.71617242066404,-1.52567909229178,0.680871998075852));
#13699=CARTESIAN_POINT('Ctrl Pts',(0.325082213976654,-1.47092890938704,
0.680973392412944));
#13700=CARTESIAN_POINT('Ctrl Pts',(12.8354863574981,-2.13063349031027,0.613986809996789));
#13701=CARTESIAN_POINT('Ctrl Pts',(11.0592740266891,-1.93586902238569,0.614841183901826));
#13702=CARTESIAN_POINT('Ctrl Pts',(6.89620783868867,-1.62958780289117,0.615922665333222));
#13703=CARTESIAN_POINT('Ctrl Pts',(2.71609101918193,-1.52912950204849,0.615919334096661));
#13704=CARTESIAN_POINT('Ctrl Pts',(0.325002675768742,-1.47440456706157,
0.616038917109795));
#13705=CARTESIAN_POINT('Ctrl Pts',(0.325002675768742,-1.47440456706157,
0.616038917109795));
#13706=CARTESIAN_POINT('Ctrl Pts',(2.71609101918193,-1.52912950204849,0.615919334096661));
#13707=CARTESIAN_POINT('Ctrl Pts',(6.89620783868867,-1.62958780289117,0.615922665333222));
#13708=CARTESIAN_POINT('Ctrl Pts',(11.0592740266891,-1.93586902238569,0.614841183901826));
#13709=CARTESIAN_POINT('Ctrl Pts',(12.8354863574981,-2.13063349031027,0.613986809996789));
#13710=CARTESIAN_POINT('Ctrl Pts',(12.8681436286308,-1.83274446434879,0.9));
#13711=CARTESIAN_POINT('Ctrl Pts',(11.0848390724976,-1.63724259846481,0.9));
#13712=CARTESIAN_POINT('Ctrl Pts',(6.90843812479705,-1.33014681916253,0.9));
#13713=CARTESIAN_POINT('Ctrl Pts',(2.72316671642812,-1.22963564084767,0.9));
#13714=CARTESIAN_POINT('Ctrl Pts',(0.331856371369203,-1.17491202960101,
0.9));
#13715=CARTESIAN_POINT('Ctrl Pts',(13.2003520234216,-1.86554403325358,-0.00671700702553119));
#13716=CARTESIAN_POINT('Ctrl Pts',(13.1894788444661,-1.85461114646479,0.200755606855839));
#13717=CARTESIAN_POINT('Ctrl Pts',(13.1786056663403,-1.84367795836273,0.40822820490283));
#13718=CARTESIAN_POINT('Ctrl Pts',(13.1677324890572,-1.83274446434879,0.615700786872884));
#13719=CARTESIAN_POINT('Ctrl Pts',(13.200220264666,-1.91338509859121,-0.00420290020003313));
#13720=CARTESIAN_POINT('Ctrl Pts',(13.1893470894366,-1.90245705934317,0.203270015787334));
#13721=CARTESIAN_POINT('Ctrl Pts',(13.1784738563058,-1.89152871992859,0.410742913234898));
#13722=CARTESIAN_POINT('Ctrl Pts',(13.1676006827814,-1.88060011874606,0.61821580043722));
#13723=CARTESIAN_POINT('Ctrl Pts',(13.1765676699515,-2.00888806967359,-0.000409897060868941));
#13724=CARTESIAN_POINT('Ctrl Pts',(13.1656896254949,-1.99796966505382,0.207063364242462));
#13725=CARTESIAN_POINT('Ctrl Pts',(13.1548115799789,-1.98705090404177,0.414536607525659));
#13726=CARTESIAN_POINT('Ctrl Pts',(13.1439334900924,-1.97613202744891,0.622009843787749));
#13727=CARTESIAN_POINT('Ctrl Pts',(13.0627995670833,-2.13884429305335,0.000475886042502645));
#13728=CARTESIAN_POINT('Ctrl Pts',(13.0518999280859,-2.12793157960824,0.207948441605934));
#13729=CARTESIAN_POINT('Ctrl Pts',(13.041000104914,-2.11701865581933,0.415420978499924));
#13730=CARTESIAN_POINT('Ctrl Pts',(13.0301002136907,-2.10610551685206,0.62289350259018));
#13731=CARTESIAN_POINT('Ctrl Pts',(12.9395973356642,-2.17103883395928,-0.00428435975826336));
#13732=CARTESIAN_POINT('Ctrl Pts',(12.9286794517625,-2.16011362679945,0.203186612960554));
#13733=CARTESIAN_POINT('Ctrl Pts',(12.9177614752639,-2.14918756369419,0.410657536673191));
#13734=CARTESIAN_POINT('Ctrl Pts',(12.9068431708026,-2.13826180183499,0.618128462699307));
#13735=CARTESIAN_POINT('Ctrl Pts',(12.8682582931239,-2.16344935299393,-0.00842301254802964));
#13736=CARTESIAN_POINT('Ctrl Pts',(12.857334548107,-2.15251107312608,0.1990469563258));
#13737=CARTESIAN_POINT('Ctrl Pts',(12.8464105706338,-2.1415724540018,0.406516897309109));
#13738=CARTESIAN_POINT('Ctrl Pts',(12.8354863574981,-2.13063349031027,0.61398680999679));
#13739=CARTESIAN_POINT('Ctrl Pts',(13.2,-1.86519007666192,-2.60208521396521E-17));
#13740=CARTESIAN_POINT('Ctrl Pts',(13.1892441622028,-1.85437516893481,0.20523361119958));
#13741=CARTESIAN_POINT('Ctrl Pts',(13.1784883252177,-1.84355996631422,0.410467206902138));
#13742=CARTESIAN_POINT('Ctrl Pts',(13.1677324890572,-1.83274446434879,0.615700786872884));
#13743=CARTESIAN_POINT('Ctrl Pts',(12.8354863574981,-2.13063349031027,0.61398680999679));
#13744=CARTESIAN_POINT('Ctrl Pts',(12.8462627343229,-2.14142441807303,0.409324567403199));
#13745=CARTESIAN_POINT('Ctrl Pts',(12.8570388818204,-2.15221501053143,0.204662297274642));
#13746=CARTESIAN_POINT('Ctrl Pts',(12.8678148030684,-2.16300527278357,2.15973072759112E-16));
#13747=CARTESIAN_POINT('Ctrl Pts',(12.868249917342,2.16344096606744,-0.0082639349430893));
#13748=CARTESIAN_POINT('Ctrl Pts',(12.8573289641336,2.15250548166836,0.19915300804817));
#13749=CARTESIAN_POINT('Ctrl Pts',(12.8464077785869,2.14156965818488,0.406569923163064));
#13750=CARTESIAN_POINT('Ctrl Pts',(12.8354863574981,2.13063349031027,0.613986809996789));
#13751=CARTESIAN_POINT('Ctrl Pts',(12.9158092820513,2.16850062662823,-0.00550483257449158));
#13752=CARTESIAN_POINT('Ctrl Pts',(12.9048922561706,2.15757374897544,0.201912774743134));
#13753=CARTESIAN_POINT('Ctrl Pts',(12.8939750281693,2.14664650750606,0.409330354360154));
#13754=CARTESIAN_POINT('Ctrl Pts',(12.8830575663678,2.13571903132675,0.616747911798467));
#13755=CARTESIAN_POINT('Ctrl Pts',(13.0132876381743,2.15534286385676,-0.00108956416640176));
#13756=CARTESIAN_POINT('Ctrl Pts',(13.002382910411,2.14442874534411,0.206329347217122));
#13757=CARTESIAN_POINT('Ctrl Pts',(12.9914779109393,2.13351435475356,0.413748232116966));
#13758=CARTESIAN_POINT('Ctrl Pts',(12.9805728576194,2.12259976690609,0.621167106093357));
#13759=CARTESIAN_POINT('Ctrl Pts',(13.1547834649542,2.05631410774027,0.001107541479323));
#13760=CARTESIAN_POINT('Ctrl Pts',(13.1439034803964,2.04540309863889,0.208527817346591));
#13761=CARTESIAN_POINT('Ctrl Pts',(13.1330234810862,2.03449182132921,0.415948079627069));
#13762=CARTESIAN_POINT('Ctrl Pts',(13.1221434051731,2.0235803832085,0.623368331037722));
#13763=CARTESIAN_POINT('Ctrl Pts',(13.2001460482598,1.93729725403583,-0.00278676680844524));
#13764=CARTESIAN_POINT('Ctrl Pts',(13.1892758011844,1.92637447722781,0.204633283810596));
#13765=CARTESIAN_POINT('Ctrl Pts',(13.1784050234814,1.91545126126866,0.412053283701094));
#13766=CARTESIAN_POINT('Ctrl Pts',(13.1675347796435,1.9045279459447,0.619473307219386));
#13767=CARTESIAN_POINT('Ctrl Pts',(13.2003436864113,1.86553565046225,-0.00655792739252892));
#13768=CARTESIAN_POINT('Ctrl Pts',(13.1894732864596,1.85460555778322,0.200861659936414));
#13769=CARTESIAN_POINT('Ctrl Pts',(13.1786028873373,1.84367516394377,0.408281231439009));
#13770=CARTESIAN_POINT('Ctrl Pts',(13.1677324890572,1.83274446434879,0.615700786872883));
#13771=CARTESIAN_POINT('Ctrl Pts',(12.8678148030684,2.16300527278357,-3.77302356024956E-17));
#13772=CARTESIAN_POINT('Ctrl Pts',(12.8570388818204,2.15221501053142,0.204662297274639));
#13773=CARTESIAN_POINT('Ctrl Pts',(12.8462627343229,2.14142441807303,0.409324567403198));
#13774=CARTESIAN_POINT('Ctrl Pts',(12.8354863574981,2.13063349031027,0.613986809996789));
#13775=CARTESIAN_POINT('Ctrl Pts',(13.1677324890572,1.83274446434879,0.615700786872883));
#13776=CARTESIAN_POINT('Ctrl Pts',(13.1784883252177,1.84355996631422,0.410467206902138));
#13777=CARTESIAN_POINT('Ctrl Pts',(13.1892441622028,1.85437516893481,0.20523361119958));
#13778=CARTESIAN_POINT('Ctrl Pts',(13.2,1.86519007666192,9.4542429440736E-17));
#13779=CARTESIAN_POINT('Ctrl Pts',(0.3318563713692,1.17491202960101,0.9));
#13780=CARTESIAN_POINT('Ctrl Pts',(2.72316671642811,1.22963564084767,0.9));
#13781=CARTESIAN_POINT('Ctrl Pts',(6.90843812479704,1.33014681916253,0.9));
#13782=CARTESIAN_POINT('Ctrl Pts',(11.0848390724976,1.63724259846481,0.9));
#13783=CARTESIAN_POINT('Ctrl Pts',(12.8681436286308,1.83274446434879,0.9));
#13784=CARTESIAN_POINT('Ctrl Pts',(0.329872740993969,1.26159263654569,0.9));
#13785=CARTESIAN_POINT('Ctrl Pts',(2.72111811994415,1.31633797570969,0.90000078069347));
#13786=CARTESIAN_POINT('Ctrl Pts',(6.90489492800774,1.41683381760594,0.90000280557396));
#13787=CARTESIAN_POINT('Ctrl Pts',(11.0774332085042,1.7238803779394,0.89999435405169));
#13788=CARTESIAN_POINT('Ctrl Pts',(12.8586523934408,1.91932043067563,0.9));
#13789=CARTESIAN_POINT('Ctrl Pts',(0.326433810179882,1.41186690836963,0.829991693349937));
#13790=CARTESIAN_POINT('Ctrl Pts',(2.71756729604703,1.46664725828863,0.829952661937692));
#13791=CARTESIAN_POINT('Ctrl Pts',(6.89876476423633,1.56711486110062,0.829953500700133));
#13792=CARTESIAN_POINT('Ctrl Pts',(11.0645720435655,1.87407163985848,0.829602081442736));
#13793=CARTESIAN_POINT('Ctrl Pts',(12.8422006781022,2.06938763738452,0.829321796184828));
#13794=CARTESIAN_POINT('Ctrl Pts',(0.325082213976652,1.47092890938703,0.680973392412944));
#13795=CARTESIAN_POINT('Ctrl Pts',(2.71617242066403,1.52567909229178,0.680871998075852));
#13796=CARTESIAN_POINT('Ctrl Pts',(6.89634818471838,1.62613750062048,0.680874066334139));
#13797=CARTESIAN_POINT('Ctrl Pts',(11.0595580661442,1.93265366192027,0.679962478070753));
#13798=CARTESIAN_POINT('Ctrl Pts',(12.8358182377562,2.12760618633201,0.679236780301187));
#13799=CARTESIAN_POINT('Ctrl Pts',(0.32500267576874,1.47440456706157,0.616038917109795));
#13800=CARTESIAN_POINT('Ctrl Pts',(2.71609101918192,1.52912950204849,0.615919334096661));
#13801=CARTESIAN_POINT('Ctrl Pts',(6.89620783868868,1.62958780289117,0.615922665333222));
#13802=CARTESIAN_POINT('Ctrl Pts',(11.0592740266891,1.93586902238569,0.614841183901826));
#13803=CARTESIAN_POINT('Ctrl Pts',(12.8354863574981,2.13063349031027,0.613986809996789));
#13804=CARTESIAN_POINT('Ctrl Pts',(12.8354863574981,2.13063349031027,0.613986809996789));
#13805=CARTESIAN_POINT('Ctrl Pts',(11.0592740266891,1.93586902238569,0.614841183901826));
#13806=CARTESIAN_POINT('Ctrl Pts',(6.89620783868868,1.62958780289117,0.615922665333222));
#13807=CARTESIAN_POINT('Ctrl Pts',(2.71609101918192,1.52912950204849,0.615919334096661));
#13808=CARTESIAN_POINT('Ctrl Pts',(0.32500267576874,1.47440456706157,0.616038917109795));
#13809=CARTESIAN_POINT('Ctrl Pts',(0.331856371879031,1.17491202961268,0.900000000000001));
#13810=CARTESIAN_POINT('Ctrl Pts',(2.72316671676804,1.22963564085583,0.9));
#13811=CARTESIAN_POINT('Ctrl Pts',(6.90843812496665,1.330146819175,0.9));
#13812=CARTESIAN_POINT('Ctrl Pts',(11.0848390724976,1.63724259846481,0.9));
#13813=CARTESIAN_POINT('Ctrl Pts',(12.8681436286308,1.83274446434879,0.9));
#13814=CARTESIAN_POINT('Ctrl Pts',(-0.00034095850043725,1.20748740317979,
-0.0065058757516861));
#13815=CARTESIAN_POINT('Ctrl Pts',(0.0105285311667133,1.19662889149835,
0.200896342313063));
#13816=CARTESIAN_POINT('Ctrl Pts',(0.0213980209804115,1.18577043337405,
0.408298563174108));
#13817=CARTESIAN_POINT('Ctrl Pts',(0.0322675109428289,1.17491202960101,
0.615700786872884));
#13818=CARTESIAN_POINT('Ctrl Pts',(-9.96670524854573E-5,1.295669506487,
-0.00190176065173685));
#13819=CARTESIAN_POINT('Ctrl Pts',(0.0107698931059531,1.28480880908357,
0.205500324005663));
#13820=CARTESIAN_POINT('Ctrl Pts',(0.0216392211477595,1.27394827585187,
0.412902429485043));
#13821=CARTESIAN_POINT('Ctrl Pts',(0.0325087822871292,1.26308766450658,
0.62030451837231));
#13822=CARTESIAN_POINT('Ctrl Pts',(0.0728623575603101,1.44853010213391,
0.00227745497540766));
#13823=CARTESIAN_POINT('Ctrl Pts',(0.0837280751164453,1.43766588856392,
0.209679530627308));
#13824=CARTESIAN_POINT('Ctrl Pts',(0.0945938325013454,1.42680163888532,
0.41708160190494));
#13825=CARTESIAN_POINT('Ctrl Pts',(0.105459512942901,1.41593747613444,0.624483681552028));
#13826=CARTESIAN_POINT('Ctrl Pts',(0.226308920038025,1.50529438233544,-0.00279245331904538));
#13827=CARTESIAN_POINT('Ctrl Pts',(0.237168779176494,1.4944331215396,0.204610074087555));
#13828=CARTESIAN_POINT('Ctrl Pts',(0.248028678199983,1.48357195724705,0.412012604182119));
#13829=CARTESIAN_POINT('Ctrl Pts',(0.258888441593434,1.47271077595937,0.619415140009235));
#13830=CARTESIAN_POINT('Ctrl Pts',(0.292428177212438,1.50698080067503,-0.00616932457891824));
#13831=CARTESIAN_POINT('Ctrl Pts',(0.303286399461314,1.49612200437087,0.201233417384176));
#13832=CARTESIAN_POINT('Ctrl Pts',(0.314144565926839,1.48526325958177,0.408636164588429));
#13833=CARTESIAN_POINT('Ctrl Pts',(0.325002675768741,1.47440456706157,0.616038917109795));
#13834=CARTESIAN_POINT('Ctrl Pts',(1.62630325872826E-19,1.20714678905882,
-9.93129189996722E-17));
#13835=CARTESIAN_POINT('Ctrl Pts',(0.0107558368367203,1.19640181653194,
0.205233592872363));
#13836=CARTESIAN_POINT('Ctrl Pts',(0.0215116738169619,1.18565689645617,
0.410467188483274));
#13837=CARTESIAN_POINT('Ctrl Pts',(0.0322675109428289,1.17491202960101,
0.615700786872884));
#13838=CARTESIAN_POINT('Ctrl Pts',(0.325002675768741,1.47440456706157,0.616038917109795));
#13839=CARTESIAN_POINT('Ctrl Pts',(0.314252226354851,1.48515559337638,0.410692606218907));
#13840=CARTESIAN_POINT('Ctrl Pts',(0.30350172143464,1.49590667092872,0.205346300540215));
#13841=CARTESIAN_POINT('Ctrl Pts',(0.292751161823635,1.50665779898694,-1.27502175484295E-16));
#13842=CARTESIAN_POINT('Ctrl Pts',(12.8678148030684,-2.16300527278356,0.));
#13843=CARTESIAN_POINT('Ctrl Pts',(12.8575947095063,-2.15224352891768,0.205346305703265));
#13844=CARTESIAN_POINT('Ctrl Pts',(12.8473746159443,-2.14148178505179,0.41069261140653));
#13845=CARTESIAN_POINT('Ctrl Pts',(12.8371545223823,-2.13072004118591,0.616038917109795));
#13846=CARTESIAN_POINT('Ctrl Pts',(8.67612692265345,-1.70561506876628,0.));
#13847=CARTESIAN_POINT('Ctrl Pts',(8.67274165808153,-1.69485332490039,0.205346305703265));
#13848=CARTESIAN_POINT('Ctrl Pts',(8.66935639350961,-1.68409158103451,0.41069261140653));
#13849=CARTESIAN_POINT('Ctrl Pts',(8.6659711289377,-1.67332983716862,0.616038917109795));
#13850=CARTESIAN_POINT('Ctrl Pts',(4.48443904223854,-1.60211086545473,0.));
#13851=CARTESIAN_POINT('Ctrl Pts',(4.48788860665674,-1.59134912158884,0.205346305703265));
#13852=CARTESIAN_POINT('Ctrl Pts',(4.49133817107494,-1.58058737772296,0.41069261140653));
#13853=CARTESIAN_POINT('Ctrl Pts',(4.49478773549313,-1.56982563385707,0.616038917109795));
#13854=CARTESIAN_POINT('Ctrl Pts',(0.292751161823634,-1.50665779898694,
0.));
#13855=CARTESIAN_POINT('Ctrl Pts',(0.303035555231945,-1.49589605512106,
0.205346305703265));
#13856=CARTESIAN_POINT('Ctrl Pts',(0.313319948640256,-1.48513431125517,
0.41069261140653));
#13857=CARTESIAN_POINT('Ctrl Pts',(0.323604342048567,-1.47437256738929,
0.616038917109795));
#13858=CARTESIAN_POINT('Origin',(0.,-1.5,0.));
#13859=CARTESIAN_POINT('Origin',(6.87409734069396,-2.22044604925031E-16,
0.9));
#13860=CARTESIAN_POINT('Ctrl Pts',(0.292751161823634,1.50665779898694,0.));
#13861=CARTESIAN_POINT('Ctrl Pts',(0.303035555231945,1.49589605512106,0.205346305703265));
#13862=CARTESIAN_POINT('Ctrl Pts',(0.313319948640256,1.48513431125517,0.41069261140653));
#13863=CARTESIAN_POINT('Ctrl Pts',(0.323604342048567,1.47437256738929,0.616038917109795));
#13864=CARTESIAN_POINT('Ctrl Pts',(4.48443904223854,1.60211086545473,0.));
#13865=CARTESIAN_POINT('Ctrl Pts',(4.48788860665674,1.59134912158884,0.205346305703265));
#13866=CARTESIAN_POINT('Ctrl Pts',(4.49133817107493,1.58058737772296,0.41069261140653));
#13867=CARTESIAN_POINT('Ctrl Pts',(4.49478773549313,1.56982563385707,0.616038917109795));
#13868=CARTESIAN_POINT('Ctrl Pts',(8.67612692265345,1.70561506876628,0.));
#13869=CARTESIAN_POINT('Ctrl Pts',(8.67274165808153,1.69485332490039,0.205346305703265));
#13870=CARTESIAN_POINT('Ctrl Pts',(8.66935639350961,1.68409158103451,0.41069261140653));
#13871=CARTESIAN_POINT('Ctrl Pts',(8.66597112893769,1.67332983716862,0.616038917109795));
#13872=CARTESIAN_POINT('Ctrl Pts',(12.8678148030684,2.16300527278356,0.));
#13873=CARTESIAN_POINT('Ctrl Pts',(12.8575947095063,2.15224352891768,0.205346305703265));
#13874=CARTESIAN_POINT('Ctrl Pts',(12.8473746159443,2.14148178505179,0.41069261140653));
#13875=CARTESIAN_POINT('Ctrl Pts',(12.8371545223823,2.13072004118591,0.616038917109795));
#13876=CARTESIAN_POINT('Origin',(13.2,2.2,0.));
#19600=UNCERTAINTY_MEASURE_WITH_UNIT(LENGTH_MEASURE(0.001),#19619,
'DISTANCE_ACCURACY_VALUE',
'Maximum model space distance between geometric entities at asserted c
onnectivities');
#19605=UNCERTAINTY_MEASURE_WITH_UNIT(LENGTH_MEASURE(0.001),#19619,
'DISTANCE_ACCURACY_VALUE',
'Maximum model space distance between geometric entities at asserted c
onnectivities');
#19613=(
GEOMETRIC_REPRESENTATION_CONTEXT(3)
GLOBAL_UNCERTAINTY_ASSIGNED_CONTEXT((#19600))
GLOBAL_UNIT_ASSIGNED_CONTEXT((#19619,#19621,#19622))
REPRESENTATION_CONTEXT('','3D')
);
#19618=(
GEOMETRIC_REPRESENTATION_CONTEXT(3)
GLOBAL_UNCERTAINTY_ASSIGNED_CONTEXT((#19605))
GLOBAL_UNIT_ASSIGNED_CONTEXT((#19619,#19621,#19622))
REPRESENTATION_CONTEXT('','3D')
);
#19619=(
LENGTH_UNIT()
NAMED_UNIT(*)
SI_UNIT(.CENTI.,.METRE.)
);
#19621=(
NAMED_UNIT(*)
PLANE_ANGLE_UNIT()
SI_UNIT($,.RADIAN.)
);
#19622=(
NAMED_UNIT(*)
SI_UNIT($,.STERADIAN.)
SOLID_ANGLE_UNIT()
);
#19630=SHAPE_DEFINITION_REPRESENTATION(#19642,#19670);
#19642=PRODUCT_DEFINITION_SHAPE('',$,#19683);
#19670=SHAPE_REPRESENTATION('',(#7475),#19613);
#19675=PRODUCT_DEFINITION_CONTEXT('part definition',#19713,'design');
#19683=PRODUCT_DEFINITION('2026-11-10-01-34-59-959',
'Lower structural shell',#19695,#19675);
#19695=PRODUCT_DEFINITION_FORMATION('',$,#19722);
#19713=APPLICATION_CONTEXT(
'Core Data for Automotive Mechanical Design Process');
#19714=PRODUCT_CONTEXT('part definition',#19713,'mechanical');
#19722=PRODUCT('2026-11-10-01-34-59-959','Lower structural shell',$,(#19714));
#19731=PRESENTATION_STYLE_ASSIGNMENT((#19739));
#19739=SURFACE_STYLE_USAGE(.BOTH.,#19747);
#19747=SURFACE_SIDE_STYLE('',(#19755));
#19755=SURFACE_STYLE_FILL_AREA(#19763);
#19763=FILL_AREA_STYLE('Structural dark blue',(#19771));
#19771=FILL_AREA_STYLE_COLOUR('Structural dark blue',#19779);
#19779=COLOUR_RGB('Structural dark blue',0.0901960784313725,0.270588235294118,
0.513725490196078);
ENDSEC;
END-ISO-10303-21;
